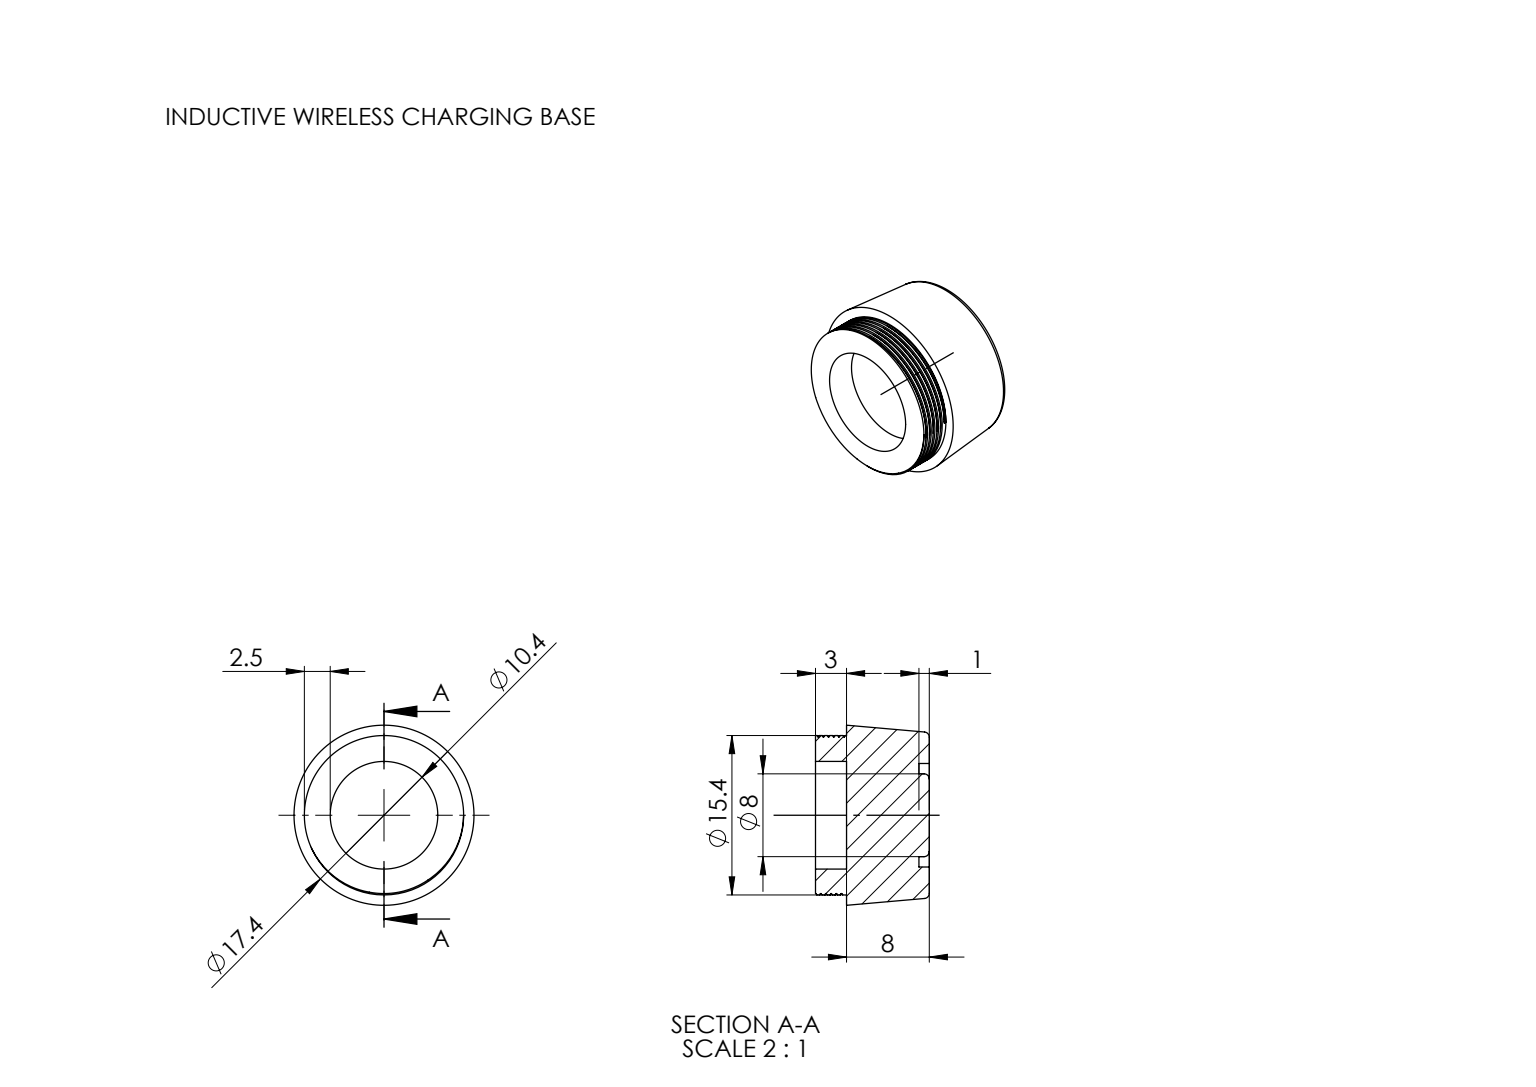
ISO-10303-21;
HEADER;
FILE_DESCRIPTION (('STEP AP214'),
    '1' );
FILE_NAME ('Inductive Wireless Charging Base.step',
    '2026-10-02T09:26:43',
    ( '' ),
    ( '' ),
    'SwSTEP 2.0',
    'SolidWorks 2026',
    '' );
FILE_SCHEMA (( 'AUTOMOTIVE_DESIGN' ));
ENDSEC;

DATA;
#217=EDGE_CURVE ( 'NONE', #101886, #26135, #31742, .T. ) ;
#447=CARTESIAN_POINT ( 'NONE',  ( 186.9479166673494603, -6.668395609140176816, -3.850000000000003642 ) ) ;
#539=ORIENTED_EDGE ( 'NONE', *, *, #28756, .T. ) ;
#549=CARTESIAN_POINT ( 'NONE',  ( 195.0435778713738557, 0.000000000000000000, 0.000000000000000000 ) ) ;
#620=DIRECTION ( 'NONE',  ( 1.000000000000000000, -0.000000000000000000, -0.000000000000000000 ) ) ;
#637=CARTESIAN_POINT ( 'NONE',  ( 184.5000000000000000, 9.429780353434619030E-16, 7.699999999999999289 ) ) ;
#712=CARTESIAN_POINT ( 'NONE',  ( 186.8229166673494603, -4.445597072760107515, 7.700000000000023270 ) ) ;
#800=CARTESIAN_POINT ( 'NONE',  ( 185.5833333333333144, -6.668395609140180369, 3.849999999999994760 ) ) ;
#962=ADVANCED_FACE ( 'NONE', ( #75850 ), #18220, .T. ) ;
#1082=ORIENTED_EDGE ( 'NONE', *, *, #3024, .T. ) ;
#1108=CARTESIAN_POINT ( 'NONE',  ( 185.4062500006828316, -8.891194145520236347, -1.633285867636356693E-15 ) ) ;
#1307=VERTEX_POINT ( 'NONE', #129199 ) ;
#1386=ORIENTED_EDGE ( 'NONE', *, *, #66111, .T. ) ;
#1422=ORIENTED_EDGE ( 'NONE', *, *, #217, .F. ) ;
#1430=FACE_OUTER_BOUND ( 'NONE', #106469, .T. ) ;
#1536=CARTESIAN_POINT ( 'NONE',  ( 184.2552083336747444, 6.551208109652275624, -3.782341765624998686 ) ) ;
#1617=DIRECTION ( 'NONE',  ( -0.9961946980917455452, -1.067350013832299517E-17, 0.08715574274765836016 ) ) ;
#1685=FACE_OUTER_BOUND ( 'NONE', #10697, .T. ) ;
#1745=CARTESIAN_POINT ( 'NONE',  ( 187.1510416670080303, 4.367472073101518859, -7.564683531249999149 ) ) ;
#1928=CARTESIAN_POINT ( 'NONE',  ( 185.4583333333333144, 4.445597072760117285, 7.699999999999999289 ) ) ;
#2069=CARTESIAN_POINT ( 'NONE',  ( 184.5000000000000000, 0.000000000000000000, 0.000000000000000000 ) ) ;
#2080=CARTESIAN_POINT ( 'NONE',  ( 187.3802083336747444, 4.367472073101515306, 7.564683531250000925 ) ) ;
#2130=ORIENTED_EDGE ( 'NONE', *, *, #61987, .T. ) ;
#2172=CARTESIAN_POINT ( 'NONE',  ( 184.3177083336747160, 4.367472073101515306, 7.564683531250000925 ) ) ;
#2331=CIRCLE ( 'NONE', #62997, 4.000000000000000000 ) ;
#2375=CARTESIAN_POINT ( 'NONE',  ( 183.9895833340161175, -4.445597072760115509, -7.700000000000001954 ) ) ;
#2389=CIRCLE ( 'NONE', #63058, 5.200000000000000178 ) ;
#2406=ORIENTED_EDGE ( 'NONE', *, *, #28810, .F. ) ;
#2444=CARTESIAN_POINT ( 'NONE',  ( 184.4999999999999432, -6.631591114337888726, -3.783919631704756092 ) ) ;
#2677=CARTESIAN_POINT ( 'NONE',  ( 184.5000000000000000, -6.267304879582558996, 4.236192450104883100 ) ) ;
#2707=CIRCLE ( 'NONE', #19432, 0.5000000000000000000 ) ;
#2714=ORIENTED_EDGE ( 'NONE', *, *, #127995, .F. ) ;
#2728=CARTESIAN_POINT ( 'NONE',  ( 187.2968750003414300, 8.734944146203032389, 5.348610694689227483E-16 ) ) ;
#2762=EDGE_CURVE ( 'NONE', #109689, #101886, #108407, .T. ) ;
#2828=CARTESIAN_POINT ( 'NONE',  ( 184.4427083336747160, -6.551208109652278289, 3.782341765624995134 ) ) ;
#2996=CARTESIAN_POINT ( 'NONE',  ( 186.0260416670080588, -6.551208109652273848, -3.782341765625003571 ) ) ;
#3024=EDGE_CURVE ( 'NONE', #82135, #52320, #124030, .T. ) ;
#3058=CARTESIAN_POINT ( 'NONE',  ( 185.7395833340161460, 4.445597072760117285, 7.699999999999999289 ) ) ;
#3067=AXIS2_PLACEMENT_3D ( 'NONE', #28494, #69048, #99815 ) ;
#3198=FACE_OUTER_BOUND ( 'NONE', #16127, .T. ) ;
#3309=VERTEX_POINT ( 'NONE', #34058 ) ;
#3320=VECTOR ( 'NONE', #123485, 1000.000000000000000 ) ;
#3378=CARTESIAN_POINT ( 'NONE',  ( 185.1718750003414016, 9.264065473108010111E-16, -7.564683531250000925 ) ) ;
#3380=CARTESIAN_POINT ( 'NONE',  ( 186.4635416670080872, -4.367472073101520635, 7.564683531249999149 ) ) ;
#3429=EDGE_CURVE ( 'NONE', #67593, #79758, #78909, .T. ) ;
#3467=CARTESIAN_POINT ( 'NONE',  ( 184.8333333333333144, 6.668395609140177704, -3.849999999999998312 ) ) ;
#3536=CYLINDRICAL_SURFACE ( 'NONE', #4210, 7.699999999999999289 ) ;
#3631=CARTESIAN_POINT ( 'NONE',  ( 185.2760416670080588, 6.551208109652274736, 3.782341765625001351 ) ) ;
#3634=CARTESIAN_POINT ( 'NONE',  ( 186.1666666666666856, -6.668395609140176816, -3.850000000000003642 ) ) ;
#3688=CARTESIAN_POINT ( 'NONE',  ( 184.4062500006828316, -8.891194145520236347, -1.633285867636356693E-15 ) ) ;
#3819=ORIENTED_EDGE ( 'NONE', *, *, #38635, .F. ) ;
#4014=CARTESIAN_POINT ( 'NONE',  ( 186.4635416670080872, -4.367472073101519747, 7.564683531249999149 ) ) ;
#4049=CARTESIAN_POINT ( 'NONE',  ( 185.9843750003414016, -8.734944146203032389, -1.604583208406767949E-15 ) ) ;
#4097=AXIS2_PLACEMENT_3D ( 'NONE', #10032, #70886, #21131 ) ;
#4210=AXIS2_PLACEMENT_3D ( 'NONE', #73550, #21906, #33647 ) ;
#4252=CARTESIAN_POINT ( 'NONE',  ( 184.5677083336747444, -4.367472073101514418, -7.564683531250002702 ) ) ;
#4305=CARTESIAN_POINT ( 'NONE',  ( 186.3593750003414016, 0.000000000000000000, 7.564683531250000925 ) ) ;
#4364=CARTESIAN_POINT ( 'NONE',  ( 184.5000000000000000, -2.986254062820097310, -7.097343634930640022 ) ) ;
#4463=DIRECTION ( 'NONE',  ( 0.000000000000000000, -1.000000000000000000, 0.000000000000000000 ) ) ;
#4514=APPLICATION_CONTEXT ( 'automotive_design' ) ;
#4558=CIRCLE ( 'NONE', #94463, 3.500000000000000000 ) ;
#4639=CARTESIAN_POINT ( 'NONE',  ( 186.7552083336747444, 6.551208109652275624, -3.782341765624998686 ) ) ;
#4640=CARTESIAN_POINT ( 'NONE',  ( 184.9635416670080588, -4.367472073101520635, 7.564683531249999149 ) ) ;
#4674=CARTESIAN_POINT ( 'NONE',  ( 185.8177083336747160, 4.367472073101515306, 7.564683531250000925 ) ) ;
#4788=CARTESIAN_POINT ( 'NONE',  ( 185.6562500006828031, 8.891194145520236347, 5.444286225454521982E-16 ) ) ;
#4904=CARTESIAN_POINT ( 'NONE',  ( 186.1510416670080588, 4.367472073101518859, -7.564683531249999149 ) ) ;
#4922=CARTESIAN_POINT ( 'NONE',  ( 184.5000000000000000, 9.429780353434619030E-16, 7.699999999999999289 ) ) ;
#4934=ADVANCED_FACE ( 'NONE', ( #116853, #38319 ), #87392, .F. ) ;
#4962=CARTESIAN_POINT ( 'NONE',  ( 185.6093750003413732, 9.264065473108010111E-16, -7.564683531250000925 ) ) ;
#5039=EDGE_LOOP ( 'NONE', ( #7533, #54215, #19907, #25528 ) ) ;
#5109=LINE ( 'NONE', #44402, #37228 ) ;
#5301=CARTESIAN_POINT ( 'NONE',  ( 186.0885416670080872, -6.551208109652273848, -3.782341765625003571 ) ) ;
#5338=CARTESIAN_POINT ( 'NONE',  ( 186.6510416670080872, 4.367472073101518859, -7.564683531249999149 ) ) ;
#5433=AXIS2_PLACEMENT_3D ( 'NONE', #62822, #113189, #13043 ) ;
#5554=CARTESIAN_POINT ( 'NONE',  ( 184.6093750003413732, 9.264065473108010111E-16, -7.564683531250000925 ) ) ;
#5599=CARTESIAN_POINT ( 'NONE',  ( 186.6093750003414016, 9.264065473108010111E-16, -7.564683531250000925 ) ) ;
#5637=ADVANCED_FACE ( 'NONE', ( #22398 ), #110953, .T. ) ;
#5816=( BOUNDED_CURVE ( )  B_SPLINE_CURVE ( 2, ( #29457, #100130, #79209, #128311, #69359, #11079, #128967 ),
 .UNSPECIFIED., .F., .F. ) 
 B_SPLINE_CURVE_WITH_KNOTS ( ( 3, 2, 2, 3 ),
 ( 0.2142857142857144681, 0.2380952380952383041, 0.2619047619047621955, 0.2857142857142859760 ),
 .UNSPECIFIED. ) 
 CURVE ( )  GEOMETRIC_REPRESENTATION_ITEM ( )  RATIONAL_B_SPLINE_CURVE ( ( 0.9999999999999988898, 0.8660254037844397068, 1.000000000000000000, 0.8660254037844387076, 1.000000000000000000, 0.8660254037844371533, 1.000000000000001554 ) ) 
 REPRESENTATION_ITEM ( '' )  );
#5905=CARTESIAN_POINT ( 'NONE',  ( 186.1145833340161175, 6.668395609140177704, -3.849999999999998312 ) ) ;
#5938=CARTESIAN_POINT ( 'NONE',  ( 186.1718750003414016, 9.264065473108010111E-16, -7.564683531250000925 ) ) ;
#5942=CARTESIAN_POINT ( 'NONE',  ( 186.0885416670080872, -6.551208109652273848, -3.782341765625003571 ) ) ;
#5974=CARTESIAN_POINT ( 'NONE',  ( 187.0677083336747160, -4.367472073101514418, -7.564683531250002702 ) ) ;
#6078=EDGE_CURVE ( 'NONE', #70723, #109689, #72930, .T. ) ;
#6192=CARTESIAN_POINT ( 'NONE',  ( 186.7135416670080872, 4.367472073101518859, -7.564683531249999149 ) ) ;
#6220=DIRECTION ( 'NONE',  ( 1.000000000000000000, -0.000000000000000000, -0.000000000000000000 ) ) ;
#6242=CARTESIAN_POINT ( 'NONE',  ( 186.8177083336747160, 4.367472073101515306, 7.564683531250000925 ) ) ;
#6511=DIRECTION ( 'NONE',  ( 1.000000000000000000, -0.000000000000000000, -0.000000000000000000 ) ) ;
#6564=CARTESIAN_POINT ( 'NONE',  ( 186.2916666666666856, 4.445597072760120838, -7.699999999999998401 ) ) ;
#6567=CARTESIAN_POINT ( 'NONE',  ( 185.7552083336747444, 6.551208109652275624, -3.782341765624998686 ) ) ;
#6572=CARTESIAN_POINT ( 'NONE',  ( 185.5312500006828031, 9.429780353434619030E-16, -7.700000000000000178 ) ) ;
#6595=CARTESIAN_POINT ( 'NONE',  ( 186.5260416670080588, -6.551208109652273848, -3.782341765625003571 ) ) ;
#6778=CARTESIAN_POINT ( 'NONE',  ( 187.1562500006828316, 8.891194145520236347, 5.444286225454521982E-16 ) ) ;
#6822=CARTESIAN_POINT ( 'NONE',  ( 185.4635416670080872, -4.367472073101519747, 7.564683531249999149 ) ) ;
#6868=DIRECTION ( 'NONE',  ( 0.4999999999999471534, 0.000000000000000000, -0.8660254037844692387 ) ) ;
#6886=VECTOR ( 'NONE', #112552, 1000.000000000000000 ) ;
#6894=CONICAL_SURFACE ( 'NONE', #50847, 8.699999999999999289, 0.08726646259971666819 ) ;
#6996=ADVANCED_FACE ( 'NONE', ( #25441 ), #102718, .F. ) ;
#7002=ADVANCED_FACE ( 'NONE', ( #53002 ), #28446, .T. ) ;
#7213=DIRECTION ( 'NONE',  ( 1.000000000000000000, -0.000000000000000000, -0.000000000000000000 ) ) ;
#7227=CARTESIAN_POINT ( 'NONE',  ( 186.7500000000000000, 9.429780353434619030E-16, -7.700000000000000178 ) ) ;
#7229=CARTESIAN_POINT ( 'NONE',  ( 185.4218750003414016, 0.000000000000000000, 7.564683531250000925 ) ) ;
#7233=AXIS2_PLACEMENT_3D ( 'NONE', #15454, #95322, #24650 ) ;
#7264=CARTESIAN_POINT ( 'NONE',  ( 185.2343750003414016, 8.734944146203032389, 5.348610694689227483E-16 ) ) ;
#7300=PRODUCT ( 'Inductive Wireless Charging Base', 'Inductive Wireless Charging Base', '', ( #106626 ) ) ;
#7328=ORIENTED_EDGE ( 'NONE', *, *, #95250, .F. ) ;
#7489=CARTESIAN_POINT ( 'NONE',  ( 187.1302083336747444, -4.367472073101514418, -7.564683531250002702 ) ) ;
#7533=ORIENTED_EDGE ( 'NONE', *, *, #8218, .F. ) ;
#7612=CARTESIAN_POINT ( 'NONE',  ( 184.7812500006828031, 0.000000000000000000, 7.700000000000000178 ) ) ;
#7681=CARTESIAN_POINT ( 'NONE',  ( 195.5000000000000000, 0.000000000000000000, 0.000000000000000000 ) ) ;
#7852=CARTESIAN_POINT ( 'NONE',  ( 186.1562500006828031, 8.891194145520236347, 5.444286225454521982E-16 ) ) ;
#7853=DIRECTION ( 'NONE',  ( 1.000000000000000000, -0.000000000000000000, -0.000000000000000000 ) ) ;
#7884=CARTESIAN_POINT ( 'NONE',  ( 184.0468750003414300, -8.734944146203032389, -1.604583208406768146E-15 ) ) ;
#7913=CARTESIAN_POINT ( 'NONE',  ( 184.9427083336747160, -6.551208109652278289, 3.782341765624995134 ) ) ;
#8132=CARTESIAN_POINT ( 'NONE',  ( 186.0885416670080872, -6.551208109652273848, -3.782341765625003571 ) ) ;
#8218=EDGE_CURVE ( 'NONE', #121663, #54095, #122867, .T. ) ;
#8279=VERTEX_POINT ( 'NONE', #111079 ) ;
#8417=SHAPE_DEFINITION_REPRESENTATION ( #77351, #18450 ) ;
#8425=CYLINDRICAL_SURFACE ( 'NONE', #64526, 7.699999999999999289 ) ;
#8518=CARTESIAN_POINT ( 'NONE',  ( 184.1302083336747160, -4.367472073101514418, -7.564683531250002702 ) ) ;
#8530=DIRECTION ( 'NONE',  ( 0.000000000000000000, -1.000000000000000000, 0.000000000000000000 ) ) ;
#8546=CARTESIAN_POINT ( 'NONE',  ( 184.5260416670080588, -6.551208109652273848, -3.782341765625003571 ) ) ;
#8563=( NAMED_UNIT ( * ) SI_UNIT ( $, .STERADIAN. ) SOLID_ANGLE_UNIT ( ) );
#8621=DIRECTION ( 'NONE',  ( 1.000000000000000000, -0.000000000000000000, -0.000000000000000000 ) ) ;
#8765=CARTESIAN_POINT ( 'NONE',  ( 185.7135416670080588, 4.367472073101518859, -7.564683531249999149 ) ) ;
#8828=AXIS2_PLACEMENT_3D ( 'NONE', #66133, #7853, #56309 ) ;
#8935=VECTOR ( 'NONE', #81638, 1000.000000000000114 ) ;
#9183=CARTESIAN_POINT ( 'NONE',  ( 183.9218750003414016, 0.000000000000000000, 7.564683531250000925 ) ) ;
#9449=AXIS2_PLACEMENT_3D ( 'NONE', #93952, #25854, #122764 ) ;
#9462=PRESENTATION_STYLE_ASSIGNMENT (( #69663 ) ) ;
#9826=CARTESIAN_POINT ( 'NONE',  ( 184.6666666666666856, -6.668395609140176816, -3.850000000000003642 ) ) ;
#9879=( NAMED_UNIT ( * ) PLANE_ANGLE_UNIT ( ) SI_UNIT ( $, .RADIAN. ) );
#9972=DIRECTION ( 'NONE',  ( 0.000000000000000000, 0.000000000000000000, 1.000000000000000000 ) ) ;
#10032=CARTESIAN_POINT ( 'NONE',  ( 184.5000000000000000, 0.000000000000000000, 0.000000000000000000 ) ) ;
#10080=CARTESIAN_POINT ( 'NONE',  ( 185.0468750003414016, -8.734944146203032389, -1.604583208406768146E-15 ) ) ;
#10277=CARTESIAN_POINT ( 'NONE',  ( 184.7083333333333428, -4.445597072760175017, -7.699999999999898037 ) ) ;
#10328=CARTESIAN_POINT ( 'NONE',  ( 187.4609375001707008, 0.000000000000000000, 7.632341765625000107 ) ) ;
#10429=CIRCLE ( 'NONE', #77334, 3.500000000000000000 ) ;
#10611=ORIENTED_EDGE ( 'NONE', *, *, #23625, .T. ) ;
#10644=CARTESIAN_POINT ( 'NONE',  ( 0.000000000000000000, 0.000000000000000000, 0.000000000000000000 ) ) ;
#10666=AXIS2_PLACEMENT_3D ( 'NONE', #58179, #68613, #117052 ) ;
#10697=EDGE_LOOP ( 'NONE', ( #109898, #53620, #81214, #33966 ) ) ;
#10776=( BOUNDED_CURVE ( )  B_SPLINE_CURVE ( 2, ( #120233, #10277, #71122, #69842, #60679, #49569, #120867 ),
 .UNSPECIFIED., .F., .F. ) 
 B_SPLINE_CURVE_WITH_KNOTS ( ( 3, 2, 2, 3 ),
 ( 0.7857142857142862535, 0.8095238095238102005, 0.8333333333333340365, 0.8571428571428578724 ),
 .UNSPECIFIED. ) 
 CURVE ( )  GEOMETRIC_REPRESENTATION_ITEM ( )  RATIONAL_B_SPLINE_CURVE ( ( 0.9999999999999968914, 0.8660254037844418162, 1.000000000000000000, 0.8660254037844387076, 1.000000000000000000, 0.8660254037844343777, 1.000000000000004441 ) ) 
 REPRESENTATION_ITEM ( '' )  );
#10901=CARTESIAN_POINT ( 'NONE',  ( 184.7395833340161460, 4.445597072760117285, 7.699999999999999289 ) ) ;
#10977=VECTOR ( 'NONE', #37893, 1000.000000000000000 ) ;
#11079=CARTESIAN_POINT ( 'NONE',  ( 186.3229166673494319, -4.445597072760092416, 7.700000000000049916 ) ) ;
#11120=ORIENTED_EDGE ( 'NONE', *, *, #103788, .F. ) ;
#11135=ORIENTED_EDGE ( 'NONE', *, *, #44217, .T. ) ;
#11175=CARTESIAN_POINT ( 'NONE',  ( 187.2500000000000000, 9.429780353434619030E-16, -7.700000000000000178 ) ) ;
#11573=CARTESIAN_POINT ( 'NONE',  ( 184.0312500006828031, 9.429780353434619030E-16, -7.700000000000000178 ) ) ;
#11909=CARTESIAN_POINT ( 'NONE',  ( 187.1302083336747444, -4.367472073101514418, -7.564683531250002702 ) ) ;
#11938=CARTESIAN_POINT ( 'NONE',  ( 187.5000000000000000, 0.000000000000000000, 0.000000000000000000 ) ) ;
#11956=CIRCLE ( 'NONE', #53720, 5.200000000000000178 ) ;
#11997=ORIENTED_EDGE ( 'NONE', *, *, #52602, .T. ) ;
#12005=ADVANCED_FACE ( 'NONE', ( #70689 ), #110610, .T. ) ;
#12203=ORIENTED_EDGE ( 'NONE', *, *, #28756, .F. ) ;
#12210=CARTESIAN_POINT ( 'NONE',  ( 185.9895833340161460, -4.445597072760115509, -7.700000000000001954 ) ) ;
#12396=CARTESIAN_POINT ( 'NONE',  ( 185.3333333333333144, 6.668395609140177704, -3.849999999999998312 ) ) ;
#12521=EDGE_CURVE ( 'NONE', #85590, #3309, #75602, .T. ) ;
#12635=CARTESIAN_POINT ( 'NONE',  ( 184.1093750003413732, 9.264065473108010111E-16, -7.564683531250000925 ) ) ;
#12681=EDGE_LOOP ( 'NONE', ( #2406, #115928, #39495, #11120 ) ) ;
#12695=MANIFOLD_SOLID_BREP ( 'Cavity1', #56137 ) ;
#12722=CARTESIAN_POINT ( 'NONE',  ( 185.4166666666666856, 6.668395609140176816, 3.850000000000000977 ) ) ;
#12787=CARTESIAN_POINT ( 'NONE',  ( 186.1927083336747160, 6.551208109652275624, -3.782341765624998686 ) ) ;
#12791=DIRECTION ( 'NONE',  ( 0.000000000000000000, 0.000000000000000000, -1.000000000000000000 ) ) ;
#12828=AXIS2_PLACEMENT_3D ( 'NONE', #77197, #105366, #117737 ) ;
#12837=CARTESIAN_POINT ( 'NONE',  ( 184.3645833340161175, -6.668395609140180369, 3.849999999999994760 ) ) ;
#12926=CARTESIAN_POINT ( 'NONE',  ( 186.5000000000000000, 0.000000000000000000, 7.700000000000000178 ) ) ;
#13043=DIRECTION ( 'NONE',  ( 0.000000000000000000, 0.000000000000000000, -1.000000000000000000 ) ) ;
#13048=CARTESIAN_POINT ( 'NONE',  ( 195.5000000000000000, 0.000000000000000000, 0.000000000000000000 ) ) ;
#13128=VECTOR ( 'NONE', #84395, 1000.000000000000000 ) ;
#13181=CARTESIAN_POINT ( 'NONE',  ( 185.4635416670080872, -4.367472073101519747, 7.564683531249999149 ) ) ;
#13235=CARTESIAN_POINT ( 'NONE',  ( 185.4895833340161175, -4.445597072760163471, -7.699999999999919353 ) ) ;
#13270=CARTESIAN_POINT ( 'NONE',  ( 184.9166666666666856, 6.668395609140176816, 3.850000000000000977 ) ) ;
#13276=CARTESIAN_POINT ( 'NONE',  ( 184.4010416670080872, -4.367472073101519747, 7.564683531249999149 ) ) ;
#13365=ORIENTED_EDGE ( 'NONE', *, *, #41805, .F. ) ;
#13440=CARTESIAN_POINT ( 'NONE',  ( 186.6093750003414016, 9.264065473108010111E-16, -7.564683531250000925 ) ) ;
#13496=CARTESIAN_POINT ( 'NONE',  ( 184.8229166673494603, -4.445597072760122614, 7.699999999999998401 ) ) ;
#13742=PLANE ( 'NONE',  #84182 ) ;
#13832=CARTESIAN_POINT ( 'NONE',  ( 185.7552083336747444, 6.551208109652275624, -3.782341765624998686 ) ) ;
#13836=CARTESIAN_POINT ( 'NONE',  ( 186.2552083336747444, 6.551208109652275624, -3.782341765624998686 ) ) ;
#13869=CARTESIAN_POINT ( 'NONE',  ( 186.0677083336747444, -4.367472073101514418, -7.564683531250002702 ) ) ;
#13916=CARTESIAN_POINT ( 'NONE',  ( 185.8229166673494319, -4.445597072760079982, 7.700000000000070344 ) ) ;
#13972=EDGE_LOOP ( 'NONE', ( #84717, #41693, #92938, #7328 ) ) ;
#14015=CARTESIAN_POINT ( 'NONE',  ( 184.5000000000000000, 0.000000000000000000, -7.699999999999999289 ) ) ;
#14025=ORIENTED_EDGE ( 'NONE', *, *, #34914, .T. ) ;
#14076=CARTESIAN_POINT ( 'NONE',  ( 184.6927083336747160, 6.551208109652275624, -3.782341765624998686 ) ) ;
#14113=AXIS2_PLACEMENT_3D ( 'NONE', #19161, #70228, #72168 ) ;
#14141=CARTESIAN_POINT ( 'NONE',  ( 186.4427083336747160, -6.551208109652278289, 3.782341765624995134 ) ) ;
#14229=( BOUNDED_CURVE ( )  B_SPLINE_CURVE ( 2, ( #60447, #108228, #100354, #68948, #28392, #108860, #18560 ),
 .UNSPECIFIED., .F., .F. ) 
 B_SPLINE_CURVE_WITH_KNOTS ( ( 3, 2, 2, 3 ),
 ( 0.4285714285714289362, 0.4523809523809527722, 0.4761904761904766081, 0.5000000000000004441 ),
 .UNSPECIFIED. ) 
 CURVE ( )  GEOMETRIC_REPRESENTATION_ITEM ( )  RATIONAL_B_SPLINE_CURVE ( ( 0.9999999999999977796, 0.8660254037844409281, 1.000000000000000000, 0.8660254037844387076, 1.000000000000000000, 0.8660254037844361541, 1.000000000000002442 ) ) 
 REPRESENTATION_ITEM ( '' )  );
#14263=CARTESIAN_POINT ( 'NONE',  ( 184.5000000000000000, -2.986254062820097310, -7.097343634930640022 ) ) ;
#14466=CARTESIAN_POINT ( 'NONE',  ( 185.5052083336747444, -6.551208109652278289, 3.782341765624995134 ) ) ;
#14469=CARTESIAN_POINT ( 'NONE',  ( 185.3385416670080872, 6.551208109652274736, 3.782341765625001351 ) ) ;
#14505=CARTESIAN_POINT ( 'NONE',  ( 185.9427083336747160, -6.551208109652278289, 3.782341765624995134 ) ) ;
#14524=CARTESIAN_POINT ( 'NONE',  ( 185.3645833340161175, -6.668395609140180369, 3.849999999999994760 ) ) ;
#14556=CARTESIAN_POINT ( 'NONE',  ( 185.7812500006828031, 0.000000000000000000, 7.700000000000000178 ) ) ;
#14718=CARTESIAN_POINT ( 'NONE',  ( 184.4843750003414016, -8.734944146203032389, -1.604583208406768146E-15 ) ) ;
#14765=CARTESIAN_POINT ( 'NONE',  ( 185.4427083336747160, -6.551208109652278289, 3.782341765624995134 ) ) ;
#14851=ORIENTED_EDGE ( 'NONE', *, *, #51179, .F. ) ;
#15054=CARTESIAN_POINT ( 'NONE',  ( 184.5000000000000000, -7.430520870378829024, -1.418378131116527108 ) ) ;
#15099=CARTESIAN_POINT ( 'NONE',  ( 186.2968750003414584, 8.734944146203032389, 5.348610694689227483E-16 ) ) ;
#15125=AXIS2_PLACEMENT_3D ( 'NONE', #39212, #79121, #69267 ) ;
#15347=DIRECTION ( 'NONE',  ( 1.000000000000000000, -0.000000000000000000, -0.000000000000000000 ) ) ;
#15362=CARTESIAN_POINT ( 'NONE',  ( 185.4010416670080588, -4.367472073101519747, 7.564683531249999149 ) ) ;
#15423=CARTESIAN_POINT ( 'NONE',  ( 185.3177083336747160, 4.367472073101515306, 7.564683531250000925 ) ) ;
#15454=CARTESIAN_POINT ( 'NONE',  ( 187.5000000000000000, 0.000000000000000000, 0.000000000000000000 ) ) ;
#15764=( BOUNDED_CURVE ( )  B_SPLINE_CURVE ( 2, ( #114067, #45339, #24397, #104244, #125176, #13916, #14556 ),
 .UNSPECIFIED., .F., .F. ) 
 B_SPLINE_CURVE_WITH_KNOTS ( ( 3, 2, 2, 3 ),
 ( 0.3571428571428574283, 0.3809523809523812643, 0.4047619047619051003, 0.4285714285714289362 ),
 .UNSPECIFIED. ) 
 CURVE ( )  GEOMETRIC_REPRESENTATION_ITEM ( )  RATIONAL_B_SPLINE_CURVE ( ( 0.9999999999999984457, 0.8660254037844402619, 1.000000000000000000, 0.8660254037844387076, 1.000000000000000000, 0.8660254037844364872, 1.000000000000002220 ) ) 
 REPRESENTATION_ITEM ( '' )  );
#15766=CARTESIAN_POINT ( 'NONE',  ( 185.0468750003414016, -8.734944146203032389, -1.604583208406768146E-15 ) ) ;
#15768=CARTESIAN_POINT ( 'NONE',  ( 184.7552083336747444, 6.551208109652275624, -3.782341765624998686 ) ) ;
#15856=CYLINDRICAL_SURFACE ( 'NONE', #119801, 7.699999999999999289 ) ;
#16013=CARTESIAN_POINT ( 'NONE',  ( 187.0468750003414300, -8.734944146203032389, -1.604583208406768146E-15 ) ) ;
#16053=CARTESIAN_POINT ( 'NONE',  ( 187.3203125005121024, 0.000000000000000000, 7.632341765625000107 ) ) ;
#16063=CARTESIAN_POINT ( 'NONE',  ( 184.8177083336747160, 4.367472073101515306, 7.564683531250000925 ) ) ;
#16127=EDGE_LOOP ( 'NONE', ( #72186, #18546, #55572, #73590 ) ) ;
#16235=EDGE_CURVE ( 'NONE', #82540, #27061, #113643, .T. ) ;
#16266=VERTEX_POINT ( 'NONE', #71255 ) ;
#16302=VECTOR ( 'NONE', #22749, 1000.000000000000000 ) ;
#16352=AXIS2_PLACEMENT_3D ( 'NONE', #121542, #92084, #111063 ) ;
#16377=LINE ( 'NONE', #49760, #90784 ) ;
#16393=CARTESIAN_POINT ( 'NONE',  ( 184.2968750003414300, 8.734944146203032389, 5.348610694689227483E-16 ) ) ;
#16396=CARTESIAN_POINT ( 'NONE',  ( 184.7968750003414584, 8.734944146203032389, 5.348610694689227483E-16 ) ) ;
#16439=ORIENTED_EDGE ( 'NONE', *, *, #59537, .T. ) ;
#16493=CARTESIAN_POINT ( 'NONE',  ( 186.0416666666666572, -4.445597072760079982, 7.700000000000070344 ) ) ;
#16544=EDGE_CURVE ( 'NONE', #82135, #97220, #55161, .T. ) ;
#16564=CARTESIAN_POINT ( 'NONE',  ( 185.1562500006828031, 8.891194145520236347, 5.444286225454521982E-16 ) ) ;
#16597=ORIENTED_EDGE ( 'NONE', *, *, #127995, .T. ) ;
#16634=AXIS2_PLACEMENT_3D ( 'NONE', #98456, #29736, #89298 ) ;
#16653=CARTESIAN_POINT ( 'NONE',  ( 185.8802083336747444, 4.367472073101515306, 7.564683531250000925 ) ) ;
#16681=ORIENTED_EDGE ( 'NONE', *, *, #19986, .T. ) ;
#16705=CARTESIAN_POINT ( 'NONE',  ( 185.2760416670080588, 6.551208109652274736, 3.782341765625001351 ) ) ;
#16770=CARTESIAN_POINT ( 'NONE',  ( 184.8645833340161175, -6.668395609140180369, 3.849999999999994760 ) ) ;
#16906=LINE ( 'NONE', #56213, #13128 ) ;
#16967=ORIENTED_EDGE ( 'NONE', *, *, #44217, .F. ) ;
#17023=CARTESIAN_POINT ( 'NONE',  ( 187.3333333333333144, 6.668395609140177704, -3.849999999999998312 ) ) ;
#17060=CARTESIAN_POINT ( 'NONE',  ( 184.6927083336747160, 6.551208109652275624, -3.782341765624998686 ) ) ;
#17088=AXIS2_PLACEMENT_3D ( 'NONE', #35751, #56016, #84842 ) ;
#17116=CARTESIAN_POINT ( 'NONE',  ( 186.2083333333333428, -4.445597072760145707, -7.699999999999951328 ) ) ;
#17152=PLANE ( 'NONE',  #67341 ) ;
#17161=EDGE_LOOP ( 'NONE', ( #107186, #36476, #78326, #49216 ) ) ;
#17287=CARTESIAN_POINT ( 'NONE',  ( 187.0052083336747444, -6.551208109652278289, 3.782341765624995134 ) ) ;
#17311=( NAMED_UNIT ( * ) SI_UNIT ( $, .STERADIAN. ) SOLID_ANGLE_UNIT ( ) );
#17430=VERTEX_POINT ( 'NONE', #63251 ) ;
#17526=CARTESIAN_POINT ( 'NONE',  ( 184.5000000000000000, 0.000000000000000000, -7.699999999999999289 ) ) ;
#17533=VERTEX_POINT ( 'NONE', #113644 ) ;
#17699=CARTESIAN_POINT ( 'NONE',  ( 187.0000000000000000, 0.000000000000000000, 7.700000000000000178 ) ) ;
#17958=CARTESIAN_POINT ( 'NONE',  ( 186.6302083336747160, -4.367472073101514418, -7.564683531250002702 ) ) ;
#17985=EDGE_CURVE ( 'NONE', #16266, #22601, #54816, .T. ) ;
#18154=CYLINDRICAL_SURFACE ( 'NONE', #58923, 7.699999999999999289 ) ;
#18157=AXIS2_PLACEMENT_3D ( 'NONE', #2069, #99647, #9972 ) ;
#18170=CARTESIAN_POINT ( 'NONE',  ( 187.0312500006828031, 9.429780353434619030E-16, -7.700000000000000178 ) ) ;
#18183=ADVANCED_FACE ( 'NONE', ( #90960 ), #73600, .T. ) ;
#18220=CYLINDRICAL_SURFACE ( 'NONE', #10666, 4.000000000000000000 ) ;
#18355=CARTESIAN_POINT ( 'NONE',  ( 186.4583333333333144, 4.445597072760117285, 7.699999999999999289 ) ) ;
#18360=DIRECTION ( 'NONE',  ( 0.000000000000000000, 0.000000000000000000, -1.000000000000000000 ) ) ;
#18383=CARTESIAN_POINT ( 'NONE',  ( 185.6510416670080303, 4.367472073101518859, -7.564683531249999149 ) ) ;
#18450=SHAPE_REPRESENTATION ( 'Inductive Wireless Charging Base', ( #108296 ), #37304 ) ;
#18546=ORIENTED_EDGE ( 'NONE', *, *, #92244, .T. ) ;
#18556=CYLINDRICAL_SURFACE ( 'NONE', #4097, 7.699999999999999289 ) ;
#18560=CARTESIAN_POINT ( 'NONE',  ( 185.7500000000000000, 9.429780353434619030E-16, -7.700000000000000178 ) ) ;
#18606=CARTESIAN_POINT ( 'NONE',  ( 186.1718750003414016, 9.264065473108010111E-16, -7.564683531250000925 ) ) ;
#18625=ORIENTED_EDGE ( 'NONE', *, *, #3429, .T. ) ;
#18668=CYLINDRICAL_SURFACE ( 'NONE', #29927, 7.699999999999999289 ) ;
#18741=CARTESIAN_POINT ( 'NONE',  ( 184.5000000000000000, 0.000000000000000000, -5.200000000000000178 ) ) ;
#18816=FACE_OUTER_BOUND ( 'NONE', #18940, .T. ) ;
#18885=DIRECTION ( 'NONE',  ( -1.000000000000000000, -0.000000000000000000, -0.000000000000000000 ) ) ;
#18940=EDGE_LOOP ( 'NONE', ( #91829, #58214, #34205, #82778, #48164, #34402, #69224, #118172, #104712, #13365, #90243, #89668, #112364, #60147, #77509 ) ) ;
#18987=CARTESIAN_POINT ( 'NONE',  ( 185.5000000000000000, 0.000000000000000000, 7.700000000000000178 ) ) ;
#19017=CARTESIAN_POINT ( 'NONE',  ( 185.5677083336747160, -4.367472073101514418, -7.564683531250002702 ) ) ;
#19026=ORIENTED_EDGE ( 'NONE', *, *, #16544, .F. ) ;
#19126=ORIENTED_EDGE ( 'NONE', *, *, #38452, .T. ) ;
#19131=CARTESIAN_POINT ( 'NONE',  ( 185.6249999999999716, -8.891194145520236347, -1.633285867636356299E-15 ) ) ;
#19161=CARTESIAN_POINT ( 'NONE',  ( 184.5000000000000000, 0.000000000000000000, 0.000000000000000000 ) ) ;
#19258=FILL_AREA_STYLE ('',( #127308 ) ) ;
#19263=ORIENTED_EDGE ( 'NONE', *, *, #217, .T. ) ;
#19371=CARTESIAN_POINT ( 'NONE',  ( 186.5000000000000000, 0.000000000000000000, 7.700000000000000178 ) ) ;
#19390=CARTESIAN_POINT ( 'NONE',  ( 186.9427083336747160, -6.551208109652278289, 3.782341765624995134 ) ) ;
#19432=AXIS2_PLACEMENT_3D ( 'NONE', #110698, #41346, #43278 ) ;
#19522=ORIENTED_EDGE ( 'NONE', *, *, #23625, .F. ) ;
#19629=AXIS2_PLACEMENT_3D ( 'NONE', #101705, #80784, #90578 ) ;
#19654=CARTESIAN_POINT ( 'NONE',  ( 184.6250000000000000, -8.891194145520236347, -1.633285867636356693E-15 ) ) ;
#19783=CIRCLE ( 'NONE', #7233, 7.699999999999999289 ) ;
#19907=ORIENTED_EDGE ( 'NONE', *, *, #42280, .T. ) ;
#19973=CARTESIAN_POINT ( 'NONE',  ( 187.5000000000000000, 0.000000000000000000, 0.000000000000000000 ) ) ;
#19986=EDGE_CURVE ( 'NONE', #67674, #17430, #103413, .T. ) ;
#20101=CARTESIAN_POINT ( 'NONE',  ( 184.5000000000000000, 6.368163355566236381E-16, 5.200000000000000178 ) ) ;
#20115=CARTESIAN_POINT ( 'NONE',  ( 186.5312500006828031, 9.429780353434619030E-16, -7.700000000000000178 ) ) ;
#20195=CARTESIAN_POINT ( 'NONE',  ( 195.5000000000000000, 4.592425496802573972E-16, 3.500000000000000000 ) ) ;
#20294=CARTESIAN_POINT ( 'NONE',  ( 184.7500000000000000, 9.429780353434619030E-16, -7.700000000000000178 ) ) ;
#20525=ADVANCED_FACE ( 'NONE', ( #36846, #87211 ), #17152, .T. ) ;
#20580=ORIENTED_EDGE ( 'NONE', *, *, #103912, .T. ) ;
#20939=CARTESIAN_POINT ( 'NONE',  ( 185.4166666666666856, 6.668395609140176816, 3.850000000000000977 ) ) ;
#20986=CARTESIAN_POINT ( 'NONE',  ( 195.5000000000000000, 0.000000000000000000, 0.000000000000000000 ) ) ;
#21121=ORIENTED_EDGE ( 'NONE', *, *, #99642, .T. ) ;
#21131=DIRECTION ( 'NONE',  ( 0.000000000000000000, 0.000000000000000000, -1.000000000000000000 ) ) ;
#21334=ADVANCED_FACE ( 'NONE', ( #63311 ), #67536, .T. ) ;
#21386=EDGE_LOOP ( 'NONE', ( #52495, #36854 ) ) ;
#21392=CARTESIAN_POINT ( 'NONE',  ( 184.8645833340161175, -6.668395609140180369, 3.849999999999994760 ) ) ;
#21492=DIRECTION ( 'NONE',  ( -1.000000000000000000, -0.000000000000000000, -0.000000000000000000 ) ) ;
#21524=ORIENTED_EDGE ( 'NONE', *, *, #41000, .T. ) ;
#21772=CARTESIAN_POINT ( 'NONE',  ( 195.5000000000000000, 0.000000000000000000, -3.500000000000000000 ) ) ;
#21850=CARTESIAN_POINT ( 'NONE',  ( 184.3385416670080872, 6.551208109652274736, 3.782341765625001351 ) ) ;
#21906=DIRECTION ( 'NONE',  ( 1.000000000000000000, -0.000000000000000000, -0.000000000000000000 ) ) ;
#22062=CARTESIAN_POINT ( 'NONE',  ( 183.9479166673494603, -6.668395609140176816, -3.850000000000003642 ) ) ;
#22366=CARTESIAN_POINT ( 'NONE',  ( 187.1666666666666856, -6.668395609140176816, -3.850000000000003642 ) ) ;
#22398=FACE_OUTER_BOUND ( 'NONE', #35561, .T. ) ;
#22442=ORIENTED_EDGE ( 'NONE', *, *, #92244, .F. ) ;
#22459=ORIENTED_EDGE ( 'NONE', *, *, #67561, .T. ) ;
#22519=DIRECTION ( 'NONE',  ( 1.000000000000000000, 0.000000000000000000, 0.000000000000000000 ) ) ;
#22582=DIRECTION ( 'NONE',  ( 0.000000000000000000, 0.000000000000000000, 1.000000000000000000 ) ) ;
#22601=VERTEX_POINT ( 'NONE', #20195 ) ;
#22646=CARTESIAN_POINT ( 'NONE',  ( 186.2343750003414016, 8.734944146203032389, 5.348610694689227483E-16 ) ) ;
#22652=CARTESIAN_POINT ( 'NONE',  ( 184.5000000000000000, 0.000000000000000000, 0.000000000000000000 ) ) ;
#22670=ORIENTED_EDGE ( 'NONE', *, *, #6078, .F. ) ;
#22707=CARTESIAN_POINT ( 'NONE',  ( 185.7812500006828031, 0.000000000000000000, 7.700000000000000178 ) ) ;
#22749=DIRECTION ( 'NONE',  ( 1.000000000000000000, -0.000000000000000000, -0.000000000000000000 ) ) ;
#22767=ORIENTED_EDGE ( 'NONE', *, *, #47594, .T. ) ;
#22943=ORIENTED_EDGE ( 'NONE', *, *, #125058, .T. ) ;
#23028=CARTESIAN_POINT ( 'NONE',  ( 186.7968750003414300, 8.734944146203032389, 5.348610694689227483E-16 ) ) ;
#23030=CARTESIAN_POINT ( 'NONE',  ( 186.7135416670080872, 4.367472073101518859, -7.564683531249999149 ) ) ;
#23080=CARTESIAN_POINT ( 'NONE',  ( 185.4062500006828031, -8.891194145520236347, -1.633285867636356299E-15 ) ) ;
#23115=CARTESIAN_POINT ( 'NONE',  ( 195.0435778713738557, 0.000000000000000000, 0.000000000000000000 ) ) ;
#23257=CARTESIAN_POINT ( 'NONE',  ( 185.9843750003414016, -8.734944146203032389, -1.604583208406768146E-15 ) ) ;
#23316=CARTESIAN_POINT ( 'NONE',  ( 185.6145833340161175, 6.668395609140177704, -3.849999999999998312 ) ) ;
#23428=AXIS2_PLACEMENT_3D ( 'NONE', #100141, #39937, #120421 ) ;
#23577=CARTESIAN_POINT ( 'NONE',  ( 186.5833333333333144, -6.668395609140180369, 3.849999999999994760 ) ) ;
#23625=EDGE_CURVE ( 'NONE', #121663, #50143, #96054, .T. ) ;
#23667=CARTESIAN_POINT ( 'NONE',  ( 186.0468750003414300, -8.734944146203032389, -1.604583208406768146E-15 ) ) ;
#23670=CARTESIAN_POINT ( 'NONE',  ( 186.4218750003414016, 0.000000000000000000, 7.564683531250000925 ) ) ;
#23693=CARTESIAN_POINT ( 'NONE',  ( 184.7500000000000000, 9.429780353434619030E-16, -7.700000000000000178 ) ) ;
#23726=EDGE_CURVE ( 'NONE', #70184, #91613, #15764, .T. ) ;
#23906=LINE ( 'NONE', #116131, #94190 ) ;
#23930=CARTESIAN_POINT ( 'NONE',  ( 184.8177083336747160, 4.367472073101515306, 7.564683531250000925 ) ) ;
#23985=CARTESIAN_POINT ( 'NONE',  ( 185.8229166673494319, -4.445597072760122614, 7.699999999999998401 ) ) ;
#24048=CARTESIAN_POINT ( 'NONE',  ( 184.5000000000000000, -7.430520870378829024, -1.418378131116527108 ) ) ;
#24195=( BOUNDED_CURVE ( )  B_SPLINE_CURVE ( 2, ( #69447, #104079, #92314, #61593, #23577, #113907, #43886 ),
 .UNSPECIFIED., .F., .F. ) 
 B_SPLINE_CURVE_WITH_KNOTS ( ( 3, 2, 2, 3 ),
 ( 0.2142857142857144681, 0.2380952380952383041, 0.2619047619047621955, 0.2857142857142859760 ),
 .UNSPECIFIED. ) 
 CURVE ( )  GEOMETRIC_REPRESENTATION_ITEM ( )  RATIONAL_B_SPLINE_CURVE ( ( 0.9999999999999988898, 0.8660254037844397068, 1.000000000000000000, 0.8660254037844387076, 1.000000000000000000, 0.8660254037844371533, 1.000000000000001554 ) ) 
 REPRESENTATION_ITEM ( '' )  );
#24311=CARTESIAN_POINT ( 'NONE',  ( 185.7135416670080588, 4.367472073101518859, -7.564683531249999149 ) ) ;
#24314=CARTESIAN_POINT ( 'NONE',  ( 184.5052083336747444, -6.551208109652278289, 3.782341765624995134 ) ) ;
#24367=CARTESIAN_POINT ( 'NONE',  ( 186.9583333333332860, 4.445597072760133273, 7.699999999999975309 ) ) ;
#24387=ADVANCED_FACE ( 'NONE', ( #71742 ), #111669, .T. ) ;
#24397=CARTESIAN_POINT ( 'NONE',  ( 185.9479166673494603, -6.668395609140176816, -3.850000000000003642 ) ) ;
#24402=CARTESIAN_POINT ( 'NONE',  ( 184.0260416670080588, -6.551208109652273848, -3.782341765625003571 ) ) ;
#24494=CARTESIAN_POINT ( 'NONE',  ( 187.5000000000000000, 6.368163355566236381E-16, 5.200000000000000178 ) ) ;
#24562=CARTESIAN_POINT ( 'NONE',  ( 185.2343750003414016, 8.734944146203032389, 5.348610694689227483E-16 ) ) ;
#24628=CARTESIAN_POINT ( 'NONE',  ( 185.5260416670080588, -6.551208109652273848, -3.782341765625003571 ) ) ;
#24650=DIRECTION ( 'NONE',  ( 0.000000000000000000, 0.000000000000000000, 1.000000000000000000 ) ) ;
#24746=ADVANCED_FACE ( 'NONE', ( #28445 ), #6894, .T. ) ;
#24847=EDGE_LOOP ( 'NONE', ( #26293, #12203, #62356, #41695 ) ) ;
#24888=DIRECTION ( 'NONE',  ( 0.000000000000000000, 0.000000000000000000, -1.000000000000000000 ) ) ;
#24954=CARTESIAN_POINT ( 'NONE',  ( 185.3385416670080872, 6.551208109652274736, 3.782341765625001351 ) ) ;
#25194=CARTESIAN_POINT ( 'NONE',  ( 186.7343750003414300, 8.734944146203032389, 5.348610694689227483E-16 ) ) ;
#25243=CARTESIAN_POINT ( 'NONE',  ( 186.9010416670080303, -4.367472073101519747, 7.564683531249999149 ) ) ;
#25303=EDGE_CURVE ( 'NONE', #97440, #36662, #29179, .T. ) ;
#25353=EDGE_LOOP ( 'NONE', ( #60289, #68706, #43931, #107555 ) ) ;
#25441=FACE_OUTER_BOUND ( 'NONE', #46842, .T. ) ;
#25458=EDGE_CURVE ( 'NONE', #52063, #55284, #69281, .T. ) ;
#25494=DIRECTION ( 'NONE',  ( 0.000000000000000000, 0.000000000000000000, -1.000000000000000000 ) ) ;
#25528=ORIENTED_EDGE ( 'NONE', *, *, #40311, .T. ) ;
#25562=AXIS2_PLACEMENT_3D ( 'NONE', #26880, #43474, #53925 ) ;
#25582=CARTESIAN_POINT ( 'NONE',  ( 185.2552083336747444, 6.551208109652275624, -3.782341765624998686 ) ) ;
#25584=CARTESIAN_POINT ( 'NONE',  ( 185.6718750003414016, 9.264065473108010111E-16, -7.564683531250000925 ) ) ;
#25617=CARTESIAN_POINT ( 'NONE',  ( 186.4010416670080588, -4.367472073101520635, 7.564683531249999149 ) ) ;
#25717=DIRECTION ( 'NONE',  ( 1.000000000000000000, 0.000000000000000000, 0.000000000000000000 ) ) ;
#25840=ADVANCED_BREP_SHAPE_REPRESENTATION ( '', ( #12695, #108296 ), #37304 ) ;
#25854=DIRECTION ( 'NONE',  ( 1.000000000000000000, 0.000000000000000000, 0.000000000000000000 ) ) ;
#25855=CARTESIAN_POINT ( 'NONE',  ( 187.4218750003414016, 0.000000000000000000, 7.564683531250000925 ) ) ;
#25915=CARTESIAN_POINT ( 'NONE',  ( 185.1927083336747160, 6.551208109652275624, -3.782341765624998686 ) ) ;
#25927=ADVANCED_FACE ( 'NONE', ( #55560 ), #105942, .T. ) ;
#25985=CIRCLE ( 'NONE', #120067, 0.4999999999999995559 ) ;
#26068=EDGE_CURVE ( 'NONE', #87604, #65296, #107227, .T. ) ;
#26076=DIRECTION ( 'NONE',  ( -1.000000000000000000, 0.000000000000000000, 0.000000000000000000 ) ) ;
#26135=VERTEX_POINT ( 'NONE', #24494 ) ;
#26254=CARTESIAN_POINT ( 'NONE',  ( 186.5416666666666856, -4.445597072760122614, 7.699999999999998401 ) ) ;
#26256=CARTESIAN_POINT ( 'NONE',  ( 186.0052083336747444, -6.551208109652278289, 3.782341765624995134 ) ) ;
#26293=ORIENTED_EDGE ( 'NONE', *, *, #17985, .F. ) ;
#26507=CARTESIAN_POINT ( 'NONE',  ( 186.1302083336747444, -4.367472073101514418, -7.564683531250002702 ) ) ;
#26558=CARTESIAN_POINT ( 'NONE',  ( 185.6927083336747160, 6.551208109652275624, -3.782341765624998686 ) ) ;
#26753=ORIENTED_EDGE ( 'NONE', *, *, #42280, .F. ) ;
#26880=CARTESIAN_POINT ( 'NONE',  ( 195.0000000000000000, 4.286263797015736595E-16, 3.500000000000000000 ) ) ;
#26893=CARTESIAN_POINT ( 'NONE',  ( 187.0833333333333144, -6.668395609140180369, 3.849999999999994760 ) ) ;
#26924=CARTESIAN_POINT ( 'NONE',  ( 185.3593750003413732, 0.000000000000000000, 7.564683531250000925 ) ) ;
#27061=VERTEX_POINT ( 'NONE', #58957 ) ;
#27102=CARTESIAN_POINT ( 'NONE',  ( 187.0729166673494603, 4.445597072760113733, -7.700000000000009948 ) ) ;
#27144=CARTESIAN_POINT ( 'NONE',  ( 183.9427083336747160, -6.551208109652278289, 3.782341765624995134 ) ) ;
#27415=EDGE_CURVE ( 'NONE', #3309, #35519, #100267, .T. ) ;
#27417=CARTESIAN_POINT ( 'NONE',  ( 184.5000000000000000, 0.000000000000000000, 0.000000000000000000 ) ) ;
#27433=CARTESIAN_POINT ( 'NONE',  ( 185.0833333333333144, -6.668395609140180369, 3.849999999999994760 ) ) ;
#27481=FACE_OUTER_BOUND ( 'NONE', #121551, .T. ) ;
#27511=CARTESIAN_POINT ( 'NONE',  ( 186.0833333333333144, -6.668395609140180369, 3.849999999999994760 ) ) ;
#27677=EDGE_CURVE ( 'NONE', #99122, #99741, #2331, .T. ) ;
#27772=CARTESIAN_POINT ( 'NONE',  ( 185.8385416670080872, 6.551208109652274736, 3.782341765625001351 ) ) ;
#28096=CARTESIAN_POINT ( 'NONE',  ( 185.1250000000000000, -8.891194145520236347, -1.633285867636356299E-15 ) ) ;
#28103=AXIS2_PLACEMENT_3D ( 'NONE', #128353, #8530, #48480 ) ;
#28185=CARTESIAN_POINT ( 'NONE',  ( 186.5833333333333144, -6.668395609140180369, 3.849999999999994760 ) ) ;
#28293=CARTESIAN_POINT ( 'NONE',  ( 184.5000000000000000, 0.000000000000000000, 0.000000000000000000 ) ) ;
#28346=CARTESIAN_POINT ( 'NONE',  ( 185.7500000000000000, 9.429780353434619030E-16, -7.700000000000000178 ) ) ;
#28392=CARTESIAN_POINT ( 'NONE',  ( 185.8333333333333144, 6.668395609140177704, -3.849999999999998312 ) ) ;
#28439=CARTESIAN_POINT ( 'NONE',  ( 186.7968750003414300, 8.734944146203032389, 5.348610694689227483E-16 ) ) ;
#28445=FACE_OUTER_BOUND ( 'NONE', #61866, .T. ) ;
#28446=TOROIDAL_SURFACE ( 'NONE', #101599, 3.500000000000000000, 0.5000000000000000000 ) ;
#28460=FACE_BOUND ( 'NONE', #63190, .T. ) ;
#28494=CARTESIAN_POINT ( 'NONE',  ( 187.5000000000000000, 0.000000000000000000, 0.000000000000000000 ) ) ;
#28703=CARTESIAN_POINT ( 'NONE',  ( 186.6145833340161175, 6.668395609140177704, -3.849999999999998312 ) ) ;
#28707=VERTEX_POINT ( 'NONE', #117714 ) ;
#28756=EDGE_CURVE ( 'NONE', #34917, #16266, #29731, .T. ) ;
#28772=CARTESIAN_POINT ( 'NONE',  ( 184.5000000000000000, 0.000000000000000000, 0.000000000000000000 ) ) ;
#28810=EDGE_CURVE ( 'NONE', #16266, #34917, #90360, .T. ) ;
#28837=CARTESIAN_POINT ( 'NONE',  ( 185.5833333333333144, -6.668395609140180369, 3.849999999999994760 ) ) ;
#28843=CARTESIAN_POINT ( 'NONE',  ( 194.5000000000000000, 0.000000000000000000, 0.000000000000000000 ) ) ;
#28868=CARTESIAN_POINT ( 'NONE',  ( 185.5260416670080588, -6.551208109652273848, -3.782341765625003571 ) ) ;
#28970=DIRECTION ( 'NONE',  ( 1.000000000000000000, -0.000000000000000000, -0.000000000000000000 ) ) ;
#29023=CYLINDRICAL_SURFACE ( 'NONE', #14113, 7.699999999999999289 ) ;
#29069=ADVANCED_FACE ( 'NONE', ( #89975 ), #18668, .T. ) ;
#29179=( BOUNDED_CURVE ( )  B_SPLINE_CURVE ( 2, ( #28346, #129144, #39473, #19131, #800, #98348, #59093 ),
 .UNSPECIFIED., .F., .F. ) 
 B_SPLINE_CURVE_WITH_KNOTS ( ( 3, 2, 2, 3 ),
 ( 0.5000000000000004441, 0.5238095238095242800, 0.5476190476190482270, 0.5714285714285719520 ),
 .UNSPECIFIED. ) 
 CURVE ( )  GEOMETRIC_REPRESENTATION_ITEM ( )  RATIONAL_B_SPLINE_CURVE ( ( 0.9999999999999974465, 0.8660254037844412611, 1.000000000000000000, 0.8660254037844387076, 1.000000000000000000, 0.8660254037844355990, 1.000000000000003109 ) ) 
 REPRESENTATION_ITEM ( '' )  );
#29244=CARTESIAN_POINT ( 'NONE',  ( 187.1093750003414016, 9.264065473108010111E-16, -7.564683531250000925 ) ) ;
#29300=CARTESIAN_POINT ( 'NONE',  ( 186.0729166673494319, 4.445597072760120838, -7.699999999999998401 ) ) ;
#29361=DIRECTION ( 'NONE',  ( 1.000000000000000000, -0.000000000000000000, -0.000000000000000000 ) ) ;
#29457=CARTESIAN_POINT ( 'NONE',  ( 186.5312500006828031, 9.429780353434619030E-16, -7.700000000000000178 ) ) ;
#29473=CARTESIAN_POINT ( 'NONE',  ( 185.0416666666666856, -4.445597072760122614, 7.699999999999998401 ) ) ;
#29716=CARTESIAN_POINT ( 'NONE',  ( 184.5052083336747444, -6.551208109652278289, 3.782341765624995134 ) ) ;
#29731=CIRCLE ( 'NONE', #102875, 4.000000000000000000 ) ;
#29736=DIRECTION ( 'NONE',  ( 1.000000000000000000, 0.000000000000000000, 0.000000000000000000 ) ) ;
#29917=CARTESIAN_POINT ( 'NONE',  ( 184.5000000000000000, 0.000000000000000000, 0.000000000000000000 ) ) ;
#29927=AXIS2_PLACEMENT_3D ( 'NONE', #38322, #40252, #110271 ) ;
#29941=CARTESIAN_POINT ( 'NONE',  ( 186.9062500006828316, -8.891194145520236347, -1.633285867636356693E-15 ) ) ;
#30319=FACE_OUTER_BOUND ( 'NONE', #58346, .T. ) ;
#30384=CARTESIAN_POINT ( 'NONE',  ( 184.8802083336747444, 4.367472073101515306, 7.564683531250000925 ) ) ;
#30642=ORIENTED_EDGE ( 'NONE', *, *, #114868, .T. ) ;
#30778=CARTESIAN_POINT ( 'NONE',  ( 184.1250000000000284, -8.891194145520236347, -1.633285867636356693E-15 ) ) ;
#30985=FACE_OUTER_BOUND ( 'NONE', #25353, .T. ) ;
#30995=EDGE_CURVE ( 'NONE', #97440, #70184, #107968, .T. ) ;
#31036=CARTESIAN_POINT ( 'NONE',  ( 185.1302083336747160, -4.367472073101514418, -7.564683531250002702 ) ) ;
#31184=CARTESIAN_POINT ( 'NONE',  ( 187.5000000000000000, -1.065442715258197248E-15, 8.699999999999999289 ) ) ;
#31236=CARTESIAN_POINT ( 'NONE',  ( 183.8645833340161175, -6.668395609140180369, 3.849999999999994760 ) ) ;
#31413=CARTESIAN_POINT ( 'NONE',  ( 184.2916666666666572, 4.445597072760120838, -7.699999999999998401 ) ) ;
#31562=CARTESIAN_POINT ( 'NONE',  ( 186.8385416670080872, 6.551208109652274736, 3.782341765625001351 ) ) ;
#31647=CARTESIAN_POINT ( 'NONE',  ( 184.5260416670080588, -6.551208109652273848, -3.782341765625003571 ) ) ;
#31654=CARTESIAN_POINT ( 'NONE',  ( 184.2135416670080588, 4.367472073101518859, -7.564683531249999149 ) ) ;
#31742=CIRCLE ( 'NONE', #125805, 5.200000000000000178 ) ;
#31814=CARTESIAN_POINT ( 'NONE',  ( 186.0000000000000000, 0.000000000000000000, 7.700000000000000178 ) ) ;
#31870=CARTESIAN_POINT ( 'NONE',  ( 187.0260416670080588, -6.551208109652273848, -3.782341765625003571 ) ) ;
#31884=ORIENTED_EDGE ( 'NONE', *, *, #12521, .F. ) ;
#32047=AXIS2_PLACEMENT_3D ( 'NONE', #58810, #29361, #69252 ) ;
#32066=CARTESIAN_POINT ( 'NONE',  ( 184.7916666666666856, 4.445597072760120838, -7.699999999999998401 ) ) ;
#32186=CARTESIAN_POINT ( 'NONE',  ( 184.4999999999999716, -7.210521358426481342, 2.491478058008155472 ) ) ;
#32478=VERTEX_POINT ( 'NONE', #62120 ) ;
#32482=CARTESIAN_POINT ( 'NONE',  ( 186.4427083336747160, -6.551208109652278289, 3.782341765624995134 ) ) ;
#32533=CARTESIAN_POINT ( 'NONE',  ( 185.4895833340161175, -4.445597072760115509, -7.700000000000001954 ) ) ;
#32635=( BOUNDED_CURVE ( )  B_SPLINE_CURVE ( 2, ( #19371, #80254, #69778, #70426, #50155, #99255, #101177 ),
 .UNSPECIFIED., .F., .F. ) 
 B_SPLINE_CURVE_WITH_KNOTS ( ( 3, 2, 2, 3 ),
 ( 0.2857142857142859760, 0.3095238095238098119, 0.3333333333333335924, 0.3571428571428574283 ),
 .UNSPECIFIED. ) 
 CURVE ( )  GEOMETRIC_REPRESENTATION_ITEM ( )  RATIONAL_B_SPLINE_CURVE ( ( 0.9999999999999984457, 0.8660254037844402619, 1.000000000000000000, 0.8660254037844387076, 1.000000000000000000, 0.8660254037844371533, 1.000000000000001554 ) ) 
 REPRESENTATION_ITEM ( '' )  );
#32867=CARTESIAN_POINT ( 'NONE',  ( 185.8802083336747444, 4.367472073101515306, 7.564683531250000925 ) ) ;
#32869=CARTESIAN_POINT ( 'NONE',  ( 187.3385416670080872, 6.551208109652274736, 3.782341765625001351 ) ) ;
#32968=EDGE_CURVE ( 'NONE', #50143, #70524, #10776, .T. ) ;
#33033=VECTOR ( 'NONE', #53964, 1000.000000000000000 ) ;
#33117=CARTESIAN_POINT ( 'NONE',  ( 186.3177083336747160, 4.367472073101515306, 7.564683531250000925 ) ) ;
#33173=CARTESIAN_POINT ( 'NONE',  ( 184.4479166673494603, -6.668395609140176816, -3.850000000000003642 ) ) ;
#33337=FACE_OUTER_BOUND ( 'NONE', #17161, .T. ) ;
#33386=( BOUNDED_CURVE ( )  B_SPLINE_CURVE ( 2, ( #73452, #24367, #113380, #54462, #55117, #103581, #123834 ),
 .UNSPECIFIED., .F., .F. ) 
 B_SPLINE_CURVE_WITH_KNOTS ( ( 3, 2, 2, 3 ),
 ( 0.1428571428571429880, 0.1666666666666668239, 0.1904761904761906322, 0.2142857142857144681 ),
 .UNSPECIFIED. ) 
 CURVE ( )  GEOMETRIC_REPRESENTATION_ITEM ( )  RATIONAL_B_SPLINE_CURVE ( ( 0.9999999999999992228, 0.8660254037844394848, 1.000000000000000000, 0.8660254037844387076, 1.000000000000000000, 0.8660254037844375974, 1.000000000000001110 ) ) 
 REPRESENTATION_ITEM ( '' )  );
#33505=CARTESIAN_POINT ( 'NONE',  ( 184.9218750003414016, 0.000000000000000000, 7.564683531250000925 ) ) ;
#33507=CARTESIAN_POINT ( 'NONE',  ( 186.3385416670080872, 6.551208109652274736, 3.782341765625001351 ) ) ;
#33647=DIRECTION ( 'NONE',  ( 0.000000000000000000, 0.000000000000000000, -1.000000000000000000 ) ) ;
#33737=CARTESIAN_POINT ( 'NONE',  ( 185.0677083336747160, -4.367472073101514418, -7.564683531250002702 ) ) ;
#33781=TOROIDAL_SURFACE ( 'NONE', #12828, 3.500000000000000000, 0.5000000000000000000 ) ;
#33793=CARTESIAN_POINT ( 'NONE',  ( 187.3177083336747444, 4.367472073101515306, 7.564683531250000925 ) ) ;
#33928=ADVANCED_FACE ( 'NONE', ( #107833 ), #18154, .T. ) ;
#33966=ORIENTED_EDGE ( 'NONE', *, *, #102227, .F. ) ;
#34058=CARTESIAN_POINT ( 'NONE',  ( 186.7812500006828031, 0.000000000000000000, 7.700000000000000178 ) ) ;
#34141=CARTESIAN_POINT ( 'NONE',  ( 186.5885416670080872, -6.551208109652273848, -3.782341765625003571 ) ) ;
#34143=CARTESIAN_POINT ( 'NONE',  ( 185.0468750003414300, -8.734944146203032389, -1.604583208406767949E-15 ) ) ;
#34205=ORIENTED_EDGE ( 'NONE', *, *, #62571, .T. ) ;
#34244=CARTESIAN_POINT ( 'NONE',  ( 184.4843750003414016, -8.734944146203032389, -1.604583208406768146E-15 ) ) ;
#34265=CARTESIAN_POINT ( 'NONE',  ( 187.5000000000000000, 0.000000000000000000, -5.200000000000000178 ) ) ;
#34350=EDGE_LOOP ( 'NONE', ( #39642, #20580, #124664, #96789 ) ) ;
#34402=ORIENTED_EDGE ( 'NONE', *, *, #85379, .F. ) ;
#34408=CARTESIAN_POINT ( 'NONE',  ( 184.6510416670080588, 4.367472073101518859, -7.564683531249999149 ) ) ;
#34457=CARTESIAN_POINT ( 'NONE',  ( 186.9427083336747160, -6.551208109652278289, 3.782341765624995134 ) ) ;
#34524=CARTESIAN_POINT ( 'NONE',  ( 184.4999999999999716, -4.098321783458930945, -6.521161088353083279 ) ) ;
#34527=ORIENTED_EDGE ( 'NONE', *, *, #125920, .T. ) ;
#34798=CARTESIAN_POINT ( 'NONE',  ( 185.9218750003414016, 0.000000000000000000, 7.564683531250000925 ) ) ;
#34800=CARTESIAN_POINT ( 'NONE',  ( 185.0052083336747444, -6.551208109652278289, 3.782341765624995134 ) ) ;
#34836=CARTESIAN_POINT ( 'NONE',  ( 187.3593750003414016, 0.000000000000000000, 7.564683531250000925 ) ) ;
#34914=EDGE_CURVE ( 'NONE', #50143, #8279, #105279, .T. ) ;
#34917=VERTEX_POINT ( 'NONE', #56792 ) ;
#35049=CARTESIAN_POINT ( 'NONE',  ( 184.3177083336747160, 4.367472073101515306, 7.564683531250000925 ) ) ;
#35105=CARTESIAN_POINT ( 'NONE',  ( 185.9427083336747160, -6.551208109652278289, 3.782341765624995134 ) ) ;
#35369=EDGE_CURVE ( 'NONE', #99741, #99122, #53125, .T. ) ;
#35432=CARTESIAN_POINT ( 'NONE',  ( 186.3802083336747444, 4.367472073101515306, 7.564683531250000925 ) ) ;
#35436=CARTESIAN_POINT ( 'NONE',  ( 185.9218750003414016, 0.000000000000000000, 7.564683531250000925 ) ) ;
#35447=CARTESIAN_POINT ( 'NONE',  ( 187.2500000000000000, 9.429780353434619030E-16, -7.700000000000000178 ) ) ;
#35466=CARTESIAN_POINT ( 'NONE',  ( 187.2343750003414016, 8.734944146203032389, 5.348610694689227483E-16 ) ) ;
#35516=CARTESIAN_POINT ( 'NONE',  ( 184.7500000000000000, 9.429780353434619030E-16, -7.700000000000000178 ) ) ;
#35519=VERTEX_POINT ( 'NONE', #107039 ) ;
#35561=EDGE_LOOP ( 'NONE', ( #47138, #34527, #40650, #100260, #53877, #98163, #120185, #97684, #124096, #66708, #94191, #92556, #10611, #36738, #126128 ) ) ;
#35650=CARTESIAN_POINT ( 'NONE',  ( 187.4218750003414016, 0.000000000000000000, 7.564683531250000925 ) ) ;
#35678=CARTESIAN_POINT ( 'NONE',  ( 187.3802083336747444, 4.367472073101515306, 7.564683531250000925 ) ) ;
#35731=CARTESIAN_POINT ( 'NONE',  ( 184.7343750003414016, 8.734944146203032389, 5.348610694689227483E-16 ) ) ;
#35751=CARTESIAN_POINT ( 'NONE',  ( 184.5000000000000000, 0.000000000000000000, 0.000000000000000000 ) ) ;
#35912=DIRECTION ( 'NONE',  ( 1.000000000000000000, -0.000000000000000000, -0.000000000000000000 ) ) ;
#36068=CARTESIAN_POINT ( 'NONE',  ( 185.8750000000000000, 8.891194145520236347, 5.444286225454521982E-16 ) ) ;
#36070=CARTESIAN_POINT ( 'NONE',  ( 184.5000000000000000, -6.267304879582558996, 4.236192450104883100 ) ) ;
#36106=CARTESIAN_POINT ( 'NONE',  ( 186.3177083336747160, 4.367472073101515306, 7.564683531250000925 ) ) ;
#36167=DIRECTION ( 'NONE',  ( 0.000000000000000000, 0.000000000000000000, -1.000000000000000000 ) ) ;
#36291=PRODUCT_DEFINITION_CONTEXT ( 'detailed design', #4514, 'design' ) ;
#36341=CARTESIAN_POINT ( 'NONE',  ( 186.9218750003414016, 0.000000000000000000, 7.564683531250000925 ) ) ;
#36380=VERTEX_POINT ( 'NONE', #6572 ) ;
#36393=CARTESIAN_POINT ( 'NONE',  ( 185.9843750003414016, -8.734944146203032389, -1.604583208406768146E-15 ) ) ;
#36476=ORIENTED_EDGE ( 'NONE', *, *, #121353, .F. ) ;
#36621=ORIENTED_EDGE ( 'NONE', *, *, #8218, .T. ) ;
#36647=FACE_OUTER_BOUND ( 'NONE', #24847, .T. ) ;
#36649=CARTESIAN_POINT ( 'NONE',  ( 185.0000000000000000, 0.000000000000000000, 7.700000000000000178 ) ) ;
#36662=VERTEX_POINT ( 'NONE', #56029 ) ;
#36698=CARTESIAN_POINT ( 'NONE',  ( 186.2812500006828031, 0.000000000000000000, 7.700000000000000178 ) ) ;
#36726=CARTESIAN_POINT ( 'NONE',  ( 186.7916666666666572, 4.445597072760120838, -7.699999999999998401 ) ) ;
#36729=CARTESIAN_POINT ( 'NONE',  ( 185.2135416670080588, 4.367472073101518859, -7.564683531249999149 ) ) ;
#36738=ORIENTED_EDGE ( 'NONE', *, *, #32968, .T. ) ;
#36760=CARTESIAN_POINT ( 'NONE',  ( 187.0260416670080588, -6.551208109652273848, -3.782341765625003571 ) ) ;
#36846=FACE_OUTER_BOUND ( 'NONE', #21386, .T. ) ;
#36854=ORIENTED_EDGE ( 'NONE', *, *, #49126, .T. ) ;
#36969=CARTESIAN_POINT ( 'NONE',  ( 185.6718750003414016, 9.264065473108010111E-16, -7.564683531250000925 ) ) ;
#37086=AXIS2_PLACEMENT_3D ( 'NONE', #102981, #22519, #62436 ) ;
#37228=VECTOR ( 'NONE', #83687, 1000.000000000000000 ) ;
#37304=( GEOMETRIC_REPRESENTATION_CONTEXT ( 3 ) GLOBAL_UNCERTAINTY_ASSIGNED_CONTEXT ( ( #99057 ) ) GLOBAL_UNIT_ASSIGNED_CONTEXT ( ( #67478, #9879, #49821 ) ) REPRESENTATION_CONTEXT ( 'NONE', 'WORKASPACE' ) );
#37372=CARTESIAN_POINT ( 'NONE',  ( 186.9583333333333428, 4.445597072760117285, 7.699999999999999289 ) ) ;
#37400=CARTESIAN_POINT ( 'NONE',  ( 184.7760416670080588, 6.551208109652274736, 3.782341765625001351 ) ) ;
#37619=CARTESIAN_POINT ( 'NONE',  ( 186.5468750003414300, -8.734944146203032389, -1.604583208406768146E-15 ) ) ;
#37698=CARTESIAN_POINT ( 'NONE',  ( 184.4999999999999716, -4.613861370277991369, 6.083321009326518869 ) ) ;
#37893=DIRECTION ( 'NONE',  ( 1.000000000000000000, -0.000000000000000000, -0.000000000000000000 ) ) ;
#37909=DIRECTION ( 'NONE',  ( 0.000000000000000000, 0.000000000000000000, -1.000000000000000000 ) ) ;
#37996=CARTESIAN_POINT ( 'NONE',  ( 187.0416666666666288, -4.445597072760122614, 7.699999999999998401 ) ) ;
#38029=CARTESIAN_POINT ( 'NONE',  ( 185.7343750003414016, 8.734944146203032389, 5.348610694689227483E-16 ) ) ;
#38053=FILL_AREA_STYLE ('',( #79277 ) ) ;
#38138=AXIS2_PLACEMENT_3D ( 'NONE', #28772, #88971, #109907 ) ;
#38262=CARTESIAN_POINT ( 'NONE',  ( 184.0677083336747160, -4.367472073101514418, -7.564683531250002702 ) ) ;
#38319=FACE_OUTER_BOUND ( 'NONE', #118677, .T. ) ;
#38322=CARTESIAN_POINT ( 'NONE',  ( 184.5000000000000000, 0.000000000000000000, 0.000000000000000000 ) ) ;
#38452=EDGE_CURVE ( 'NONE', #55284, #70524, #44080, .T. ) ;
#38572=DIRECTION ( 'NONE',  ( 0.000000000000000000, 0.000000000000000000, -1.000000000000000000 ) ) ;
#38635=EDGE_CURVE ( 'NONE', #36662, #53828, #82700, .T. ) ;
#38670=CARTESIAN_POINT ( 'NONE',  ( 185.7083333333333428, -4.445597072760115509, -7.700000000000001954 ) ) ;
#38727=SHAPE_REPRESENTATION_RELATIONSHIP ( 'NONE' , 'NONE' ,  #18450, #25840 ) ;
#39012=ADVANCED_FACE ( 'NONE', ( #30319 ), #29023, .T. ) ;
#39142=CARTESIAN_POINT ( 'NONE',  ( 186.2395833340161460, 4.445597072760117285, 7.699999999999999289 ) ) ;
#39170=VERTEX_POINT ( 'NONE', #123815 ) ;
#39212=CARTESIAN_POINT ( 'NONE',  ( 195.0000000000000000, 0.000000000000000000, 0.000000000000000000 ) ) ;
#39323=CARTESIAN_POINT ( 'NONE',  ( 184.5833333333333144, -6.668395609140180369, 3.849999999999994760 ) ) ;
#39349=CARTESIAN_POINT ( 'NONE',  ( 185.4843750003414016, -8.734944146203032389, -1.604583208406767949E-15 ) ) ;
#39473=CARTESIAN_POINT ( 'NONE',  ( 185.6666666666666856, -6.668395609140176816, -3.850000000000003642 ) ) ;
#39495=ORIENTED_EDGE ( 'NONE', *, *, #102895, .F. ) ;
#39529=EDGE_CURVE ( 'NONE', #41594, #32478, #87180, .T. ) ;
#39540=ORIENTED_EDGE ( 'NONE', *, *, #80486, .F. ) ;
#39642=ORIENTED_EDGE ( 'NONE', *, *, #27677, .T. ) ;
#39724=CARTESIAN_POINT ( 'NONE',  ( 187.3593750003414016, 0.000000000000000000, 7.564683531250000925 ) ) ;
#39777=CARTESIAN_POINT ( 'NONE',  ( 187.1145833340161175, 6.668395609140177704, -3.849999999999998312 ) ) ;
#39937=DIRECTION ( 'NONE',  ( 1.000000000000000000, 0.000000000000000000, 0.000000000000000000 ) ) ;
#39988=EDGE_CURVE ( 'NONE', #28707, #58259, #91863, .T. ) ;
#40093=EDGE_LOOP ( 'NONE', ( #3819, #30642, #47044, #26753 ) ) ;
#40190=CARTESIAN_POINT ( 'NONE',  ( 183.9635416670080872, -4.367472073101519747, 7.564683531249999149 ) ) ;
#40198=CIRCLE ( 'NONE', #113335, 5.000000000000000000 ) ;
#40252=DIRECTION ( 'NONE',  ( 1.000000000000000000, -0.000000000000000000, -0.000000000000000000 ) ) ;
#40311=EDGE_CURVE ( 'NONE', #36380, #54095, #117824, .T. ) ;
#40352=CARTESIAN_POINT ( 'NONE',  ( 187.1510416670080303, 4.367472073101518859, -7.564683531249999149 ) ) ;
#40390=DIRECTION ( 'NONE',  ( 1.000000000000000000, -0.000000000000000000, -0.000000000000000000 ) ) ;
#40635=EDGE_CURVE ( 'NONE', #22601, #44517, #10429, .T. ) ;
#40650=ORIENTED_EDGE ( 'NONE', *, *, #73518, .T. ) ;
#40768=DIRECTION ( 'NONE',  ( 0.000000000000000000, 0.000000000000000000, 1.000000000000000000 ) ) ;
#40856=CARTESIAN_POINT ( 'NONE',  ( 185.0052083336747444, -6.551208109652278289, 3.782341765624995134 ) ) ;
#40884=ADVANCED_FACE ( 'NONE', ( #54952 ), #45795, .F. ) ;
#40909=ORIENTED_EDGE ( 'NONE', *, *, #40635, .T. ) ;
#41000=EDGE_CURVE ( 'NONE', #97220, #28707, #115134, .T. ) ;
#41006=ORIENTED_EDGE ( 'NONE', *, *, #126863, .F. ) ;
#41030=( BOUNDED_CURVE ( )  B_SPLINE_CURVE ( 2, ( #115397, #44774, #106258, #16564, #96419, #45416, #65018 ),
 .UNSPECIFIED., .F., .F. ) 
 B_SPLINE_CURVE_WITH_KNOTS ( ( 3, 2, 2, 3 ),
 ( 0.5714285714285719520, 0.5952380952380957879, 0.6190476190476195129, 0.6428571428571433488 ),
 .UNSPECIFIED. ) 
 CURVE ( )  GEOMETRIC_REPRESENTATION_ITEM ( )  RATIONAL_B_SPLINE_CURVE ( ( 0.9999999999999968914, 0.8660254037844418162, 1.000000000000000000, 0.8660254037844387076, 1.000000000000000000, 0.8660254037844361541, 1.000000000000002442 ) ) 
 REPRESENTATION_ITEM ( '' )  );
#41067=CARTESIAN_POINT ( 'NONE',  ( 185.0312500006828031, 9.429780353434619030E-16, -7.700000000000000178 ) ) ;
#41241=CARTESIAN_POINT ( 'NONE',  ( 184.4166666666666856, 6.668395609140176816, 3.850000000000000977 ) ) ;
#41261=( BOUNDED_CURVE ( )  B_SPLINE_CURVE ( 2, ( #36698, #107347, #97525, #7852, #5905, #45868, #116520 ),
 .UNSPECIFIED., .F., .F. ) 
 B_SPLINE_CURVE_WITH_KNOTS ( ( 3, 2, 2, 3 ),
 ( 0.2857142857142859760, 0.3095238095238098119, 0.3333333333333335924, 0.3571428571428574283 ),
 .UNSPECIFIED. ) 
 CURVE ( )  GEOMETRIC_REPRESENTATION_ITEM ( )  RATIONAL_B_SPLINE_CURVE ( ( 0.9999999999999984457, 0.8660254037844402619, 1.000000000000000000, 0.8660254037844387076, 1.000000000000000000, 0.8660254037844371533, 1.000000000000001554 ) ) 
 REPRESENTATION_ITEM ( '' )  );
#41291=DIRECTION ( 'NONE',  ( 1.000000000000000000, 0.000000000000000000, 0.000000000000000000 ) ) ;
#41346=DIRECTION ( 'NONE',  ( 0.000000000000000000, -1.000000000000000000, 0.000000000000000000 ) ) ;
#41501=CARTESIAN_POINT ( 'NONE',  ( 184.5468750003414300, -8.734944146203032389, -1.604583208406768146E-15 ) ) ;
#41594=VERTEX_POINT ( 'NONE', #82080 ) ;
#41693=ORIENTED_EDGE ( 'NONE', *, *, #80341, .T. ) ;
#41695=ORIENTED_EDGE ( 'NONE', *, *, #40635, .F. ) ;
#41703=CARTESIAN_POINT ( 'NONE',  ( 187.1093750003414016, 9.264065473108010111E-16, -7.564683531250000925 ) ) ;
#41764=DIRECTION ( 'NONE',  ( -1.000000000000000000, -0.000000000000000000, -0.000000000000000000 ) ) ;
#41805=EDGE_CURVE ( 'NONE', #91613, #36380, #127038, .T. ) ;
#41818=LINE ( 'NONE', #81709, #63026 ) ;
#41883=CARTESIAN_POINT ( 'NONE',  ( 184.7083333333333144, -4.445597072760115509, -7.700000000000001954 ) ) ;
#42114=CIRCLE ( 'NONE', #115224, 5.000000000000000000 ) ;
#42214=CARTESIAN_POINT ( 'NONE',  ( 185.2916666666666572, 4.445597072760072876, -7.700000000000080114 ) ) ;
#42280=EDGE_CURVE ( 'NONE', #53828, #36380, #16377, .T. ) ;
#42320=DIRECTION ( 'NONE',  ( 0.000000000000000000, 0.000000000000000000, -1.000000000000000000 ) ) ;
#42333=CARTESIAN_POINT ( 'NONE',  ( 184.1979166673494603, 6.668395609140176816, 3.850000000000000977 ) ) ;
#42481=DIRECTION ( 'NONE',  ( 1.000000000000000000, -0.000000000000000000, -0.000000000000000000 ) ) ;
#42521=ORIENTED_EDGE ( 'NONE', *, *, #64751, .F. ) ;
#42567=VECTOR ( 'NONE', #28970, 1000.000000000000000 ) ;
#42691=CARTESIAN_POINT ( 'NONE',  ( 187.2552083336747444, 6.551208109652275624, -3.782341765624998686 ) ) ;
#42694=CARTESIAN_POINT ( 'NONE',  ( 186.9218750003414016, 0.000000000000000000, 7.564683531250000925 ) ) ;
#42768=CARTESIAN_POINT ( 'NONE',  ( 187.5000000000000000, 0.000000000000000000, -7.699999999999999289 ) ) ;
#42774=ORIENTED_EDGE ( 'NONE', *, *, #84262, .T. ) ;
#42874=CARTESIAN_POINT ( 'NONE',  ( 184.5000000000000000, 0.000000000000000000, 0.000000000000000000 ) ) ;
#42947=CARTESIAN_POINT ( 'NONE',  ( 185.8593750003413732, 0.000000000000000000, 7.564683531250000925 ) ) ;
#43006=CARTESIAN_POINT ( 'NONE',  ( 185.6562500006828316, 8.891194145520236347, 5.444286225454521982E-16 ) ) ;
#43196=ORIENTED_EDGE ( 'NONE', *, *, #23726, .T. ) ;
#43278=DIRECTION ( 'NONE',  ( 0.000000000000000000, 0.000000000000000000, -1.000000000000000000 ) ) ;
#43300=ORIENTED_EDGE ( 'NONE', *, *, #69291, .F. ) ;
#43325=CARTESIAN_POINT ( 'NONE',  ( 184.7135416670080872, 4.367472073101518859, -7.564683531249999149 ) ) ;
#43327=CARTESIAN_POINT ( 'NONE',  ( 186.3802083336747444, 4.367472073101515306, 7.564683531250000925 ) ) ;
#43474=DIRECTION ( 'NONE',  ( 0.000000000000000000, 1.000000000000000000, -1.224646799147353207E-16 ) ) ;
#43580=CARTESIAN_POINT ( 'NONE',  ( 185.1510416670080872, 4.367472073101518859, -7.564683531249999149 ) ) ;
#43584=CARTESIAN_POINT ( 'NONE',  ( 186.0000000000000000, 0.000000000000000000, 7.700000000000000178 ) ) ;
#43620=ORIENTED_EDGE ( 'NONE', *, *, #2762, .T. ) ;
#43636=CARTESIAN_POINT ( 'NONE',  ( 185.5729166673494319, 4.445597072760120838, -7.699999999999998401 ) ) ;
#43690=AXIS2_PLACEMENT_3D ( 'NONE', #125547, #26076, #76464 ) ;
#43798=CARTESIAN_POINT ( 'NONE',  ( 187.4609375001707008, 0.000000000000000000, 7.632341765625000107 ) ) ;
#43886=CARTESIAN_POINT ( 'NONE',  ( 186.5000000000000000, 0.000000000000000000, 7.700000000000000178 ) ) ;
#43931=ORIENTED_EDGE ( 'NONE', *, *, #27415, .T. ) ;
#43938=CARTESIAN_POINT ( 'NONE',  ( 194.5000000000000000, 0.000000000000000000, 0.000000000000000000 ) ) ;
#43961=CARTESIAN_POINT ( 'NONE',  ( 185.7968750003414300, 8.734944146203032389, 5.348610694689227483E-16 ) ) ;
#44080=B_SPLINE_CURVE_WITH_KNOTS ( 'NONE', 3,
 ( #47520, #87423, #127368, #37698, #77599, #67789, #97890, #91300, #110926, #109660, #59935, #71026 ),
 .UNSPECIFIED., .F., .F.,
 ( 4, 2, 2, 2, 2, 4 ),
 ( 0.000000000000000000, 0.001866281188413360234, 0.003732562376826720468, 0.005598843565240080485, 0.006531984159446760710, 0.007465124753653440935 ),
 .UNSPECIFIED. ) ;
#44172=DIRECTION ( 'NONE',  ( 1.000000000000000000, 0.000000000000000000, 0.000000000000000000 ) ) ;
#44192=CARTESIAN_POINT ( 'NONE',  ( 185.9427083336747160, -6.551208109652278289, 3.782341765624995134 ) ) ;
#44198=VECTOR ( 'NONE', #85389, 1000.000000000000000 ) ;
#44217=EDGE_CURVE ( 'NONE', #86499, #58259, #45593, .T. ) ;
#44248=CARTESIAN_POINT ( 'NONE',  ( 186.5677083336747160, -4.367472073101514418, -7.564683531250002702 ) ) ;
#44286=ORIENTED_EDGE ( 'NONE', *, *, #112824, .T. ) ;
#44402=CARTESIAN_POINT ( 'NONE',  ( 187.5000000000000000, 0.000000000000000000, -8.699999999999999289 ) ) ;
#44455=CARTESIAN_POINT ( 'NONE',  ( 184.5000000000000000, -7.430520870378829024, -1.418378131116527108 ) ) ;
#44517=VERTEX_POINT ( 'NONE', #21772 ) ;
#44599=CARTESIAN_POINT ( 'NONE',  ( 186.6302083336747160, -4.367472073101514418, -7.564683531250002702 ) ) ;
#44748=CARTESIAN_POINT ( 'NONE',  ( 185.5729166673494603, 4.445597072760072876, -7.700000000000080114 ) ) ;
#44774=CARTESIAN_POINT ( 'NONE',  ( 185.2395833340161460, 4.445597072760175905, 7.699999999999896261 ) ) ;
#44861=CARTESIAN_POINT ( 'NONE',  ( 184.4427083336747160, -6.551208109652278289, 3.782341765624995134 ) ) ;
#44915=CARTESIAN_POINT ( 'NONE',  ( 186.7343750003414300, 8.734944146203032389, 5.348610694689227483E-16 ) ) ;
#44981=CARTESIAN_POINT ( 'NONE',  ( 184.4999999999999716, -7.141846329728243958, -2.638575396834020648 ) ) ;
#44988=ORIENTED_EDGE ( 'NONE', *, *, #102227, .T. ) ;
#45060=ORIENTED_EDGE ( 'NONE', *, *, #35369, .F. ) ;
#45202=LINE ( 'NONE', #83816, #88483 ) ;
#45224=CYLINDRICAL_SURFACE ( 'NONE', #54323, 5.000000000000000000 ) ;
#45247=CARTESIAN_POINT ( 'NONE',  ( 186.0052083336747444, -6.551208109652278289, 3.782341765624995134 ) ) ;
#45287=CARTESIAN_POINT ( 'NONE',  ( 186.6093750003414016, 9.264065473108010111E-16, -7.564683531250000925 ) ) ;
#45339=CARTESIAN_POINT ( 'NONE',  ( 185.9895833340161175, -4.445597072760145707, -7.699999999999951328 ) ) ;
#45392=CARTESIAN_POINT ( 'NONE',  ( 185.7812500006828031, 0.000000000000000000, 7.700000000000000178 ) ) ;
#45416=CARTESIAN_POINT ( 'NONE',  ( 185.0729166673495172, 4.445597072760072876, -7.700000000000080114 ) ) ;
#45484=CARTESIAN_POINT ( 'NONE',  ( 187.3906250003414016, 0.000000000000000000, 7.700000000000000178 ) ) ;
#45510=CARTESIAN_POINT ( 'NONE',  ( 184.8593750003413732, 0.000000000000000000, 7.564683531250000925 ) ) ;
#45564=CARTESIAN_POINT ( 'NONE',  ( 184.9843750003414016, -8.734944146203032389, -1.604583208406768146E-15 ) ) ;
#45593=LINE ( 'NONE', #95969, #3320 ) ;
#45795=PLANE ( 'NONE',  #128082 ) ;
#45868=CARTESIAN_POINT ( 'NONE',  ( 186.0729166673494603, 4.445597072760091528, -7.700000000000049916 ) ) ;
#45892=CARTESIAN_POINT ( 'NONE',  ( 184.8385416670080872, 6.551208109652274736, 3.782341765625001351 ) ) ;
#45895=CARTESIAN_POINT ( 'NONE',  ( 185.4635416670080872, -4.367472073101520635, 7.564683531249999149 ) ) ;
#45933=CARTESIAN_POINT ( 'NONE',  ( 186.5677083336747160, -4.367472073101514418, -7.564683531250002702 ) ) ;
#45988=CARTESIAN_POINT ( 'NONE',  ( 184.5000000000000000, 0.000000000000000000, 0.000000000000000000 ) ) ;
#46124=ADVANCED_FACE ( 'NONE', ( #3198 ), #103324, .T. ) ;
#46134=CARTESIAN_POINT ( 'NONE',  ( 186.6718750003414016, 9.264065473108010111E-16, -7.564683531250000925 ) ) ;
#46190=CARTESIAN_POINT ( 'NONE',  ( 186.6927083336747160, 6.551208109652275624, -3.782341765624998686 ) ) ;
#46466=ADVANCED_FACE ( 'NONE', ( #90097 ), #50843, .F. ) ;
#46515=CARTESIAN_POINT ( 'NONE',  ( 186.0416666666666856, -4.445597072760122614, 7.699999999999998401 ) ) ;
#46517=CARTESIAN_POINT ( 'NONE',  ( 186.1718750003414016, 9.264065473108010111E-16, -7.564683531250000925 ) ) ;
#46548=CARTESIAN_POINT ( 'NONE',  ( 186.4427083336747160, -6.551208109652278289, 3.782341765624995134 ) ) ;
#46562=AXIS2_PLACEMENT_3D ( 'NONE', #84829, #56640, #104470 ) ;
#46791=CARTESIAN_POINT ( 'NONE',  ( 185.2968750003414300, 8.734944146203032389, 5.348610694689227483E-16 ) ) ;
#46842=EDGE_LOOP ( 'NONE', ( #86111, #86616, #1422, #52560 ) ) ;
#47034=ADVANCED_FACE ( 'NONE', ( #55027 ), #45224, .F. ) ;
#47044=ORIENTED_EDGE ( 'NONE', *, *, #41805, .T. ) ;
#47088=DIRECTION ( 'NONE',  ( 1.000000000000000000, 0.000000000000000000, 0.000000000000000000 ) ) ;
#47108=CARTESIAN_POINT ( 'NONE',  ( 185.1666666666666856, -6.668395609140176816, -3.850000000000003642 ) ) ;
#47116=ORIENTED_EDGE ( 'NONE', *, *, #3429, .F. ) ;
#47138=ORIENTED_EDGE ( 'NONE', *, *, #25458, .F. ) ;
#47185=CARTESIAN_POINT ( 'NONE',  ( 186.6250000000000284, -8.891194145520236347, -1.633285867636356693E-15 ) ) ;
#47187=CARTESIAN_POINT ( 'NONE',  ( 185.3802083336747444, 4.367472073101515306, 7.564683531250000925 ) ) ;
#47215=CARTESIAN_POINT ( 'NONE',  ( 184.7343750003414016, 8.734944146203032389, 5.348610694689227483E-16 ) ) ;
#47237=PRESENTATION_STYLE_ASSIGNMENT (( #107432 ) ) ;
#47435=CARTESIAN_POINT ( 'NONE',  ( 187.0885416670080872, -6.551208109652273848, -3.782341765625003571 ) ) ;
#47520=CARTESIAN_POINT ( 'NONE',  ( 184.5000000000000000, -6.267304879582558996, 4.236192450104883100 ) ) ;
#47541=CARTESIAN_POINT ( 'NONE',  ( 194.5000000000000000, 0.000000000000000000, -5.000000000000000000 ) ) ;
#47594=EDGE_CURVE ( 'NONE', #108189, #52320, #100103, .T. ) ;
#47629=DIRECTION ( 'NONE',  ( 0.000000000000000000, 0.000000000000000000, -1.000000000000000000 ) ) ;
#47702=EDGE_LOOP ( 'NONE', ( #47116, #73659, #82972, #41006 ) ) ;
#47836=CARTESIAN_POINT ( 'NONE',  ( 186.2083333333333144, -4.445597072760115509, -7.700000000000001954 ) ) ;
#48082=CARTESIAN_POINT ( 'NONE',  ( 185.5052083336747444, -6.551208109652278289, 3.782341765624995134 ) ) ;
#48164=ORIENTED_EDGE ( 'NONE', *, *, #16235, .F. ) ;
#48239=DIRECTION ( 'NONE',  ( -1.000000000000000000, 0.000000000000000000, 0.000000000000000000 ) ) ;
#48348=CARTESIAN_POINT ( 'NONE',  ( 194.5000000000000000, 6.123233995736766282E-16, 5.000000000000000000 ) ) ;
#48372=ADVANCED_FACE ( 'NONE', ( #71630 ), #3536, .T. ) ;
#48463=CARTESIAN_POINT ( 'NONE',  ( 185.7916666666666572, 4.445597072760120838, -7.699999999999998401 ) ) ;
#48480=DIRECTION ( 'NONE',  ( 0.000000000000000000, 0.000000000000000000, -1.000000000000000000 ) ) ;
#48538=DIRECTION ( 'NONE',  ( 0.000000000000000000, 0.000000000000000000, -1.000000000000000000 ) ) ;
#48602=LINE ( 'NONE', #128467, #42567 ) ;
#48727=CARTESIAN_POINT ( 'NONE',  ( 184.7135416670080872, 4.367472073101518859, -7.564683531249999149 ) ) ;
#48941=CARTESIAN_POINT ( 'NONE',  ( 186.4895833340161175, -4.445597072760115509, -7.700000000000001954 ) ) ;
#49047=CARTESIAN_POINT ( 'NONE',  ( 184.5312500006828031, 9.429780353434619030E-16, -7.700000000000000178 ) ) ;
#49095=EDGE_LOOP ( 'NONE', ( #124256, #56400, #43620, #67947 ) ) ;
#49126=EDGE_CURVE ( 'NONE', #109569, #17430, #125041, .T. ) ;
#49131=CARTESIAN_POINT ( 'NONE',  ( 184.2135416670080588, 4.367472073101518859, -7.564683531249999149 ) ) ;
#49164=CARTESIAN_POINT ( 'NONE',  ( 184.5677083336747444, -4.367472073101514418, -7.564683531250002702 ) ) ;
#49216=ORIENTED_EDGE ( 'NONE', *, *, #52059, .F. ) ;
#49363=AXIS2_PLACEMENT_3D ( 'NONE', #23115, #74159, #83957 ) ;
#49380=CARTESIAN_POINT ( 'NONE',  ( 185.0885416670080872, -6.551208109652273848, -3.782341765625003571 ) ) ;
#49386=CARTESIAN_POINT ( 'NONE',  ( 187.5000000000000000, 0.000000000000000000, 0.000000000000000000 ) ) ;
#49569=CARTESIAN_POINT ( 'NONE',  ( 184.5416666666666572, -4.445597072760039126, 7.700000000000142286 ) ) ;
#49591=CARTESIAN_POINT ( 'NONE',  ( 187.1562500006828316, 8.891194145520236347, 5.444286225454521982E-16 ) ) ;
#49640=CARTESIAN_POINT ( 'NONE',  ( 186.6562500006828031, 8.891194145520236347, 5.444286225454521982E-16 ) ) ;
#49668=AXIS2_PLACEMENT_3D ( 'NONE', #54336, #55624, #64791 ) ;
#49760=CARTESIAN_POINT ( 'NONE',  ( 184.5000000000000000, 0.000000000000000000, -7.699999999999999289 ) ) ;
#49777=CARTESIAN_POINT ( 'NONE',  ( 184.3333333333333144, 6.668395609140177704, -3.849999999999998312 ) ) ;
#49821=( NAMED_UNIT ( * ) SI_UNIT ( $, .STERADIAN. ) SOLID_ANGLE_UNIT ( ) );
#49959=VECTOR ( 'NONE', #125481, 1000.000000000000000 ) ;
#50005=EDGE_LOOP ( 'NONE', ( #22442, #79368, #2130, #16439 ) ) ;
#50029=CARTESIAN_POINT ( 'NONE',  ( 184.2968750003414300, 8.734944146203032389, 5.348610694689227483E-16 ) ) ;
#50143=VERTEX_POINT ( 'NONE', #23693 ) ;
#50155=CARTESIAN_POINT ( 'NONE',  ( 186.3333333333333144, 6.668395609140177704, -3.849999999999998312 ) ) ;
#50232=CARTESIAN_POINT ( 'NONE',  ( 187.0729166673494319, 4.445597072760120838, -7.699999999999998401 ) ) ;
#50457=CARTESIAN_POINT ( 'NONE',  ( 186.9479166673494603, -6.668395609140176816, -3.850000000000003642 ) ) ;
#50843=CYLINDRICAL_SURFACE ( 'NONE', #123196, 5.200000000000000178 ) ;
#50847=AXIS2_PLACEMENT_3D ( 'NONE', #49386, #89289, #80117 ) ;
#50865=CARTESIAN_POINT ( 'NONE',  ( 185.9062500006828316, -8.891194145520236347, -1.633285867636356693E-15 ) ) ;
#50971=CARTESIAN_POINT ( 'NONE',  ( 194.5000000000000000, 6.123233995736766282E-16, 5.000000000000000000 ) ) ;
#51060=CARTESIAN_POINT ( 'NONE',  ( 184.1666666666666856, -6.668395609140176816, -3.850000000000003642 ) ) ;
#51062=VECTOR ( 'NONE', #620, 1000.000000000000000 ) ;
#51135=CIRCLE ( 'NONE', #86610, 8.040022453829767102 ) ;
#51179=EDGE_CURVE ( 'NONE', #67593, #41594, #100034, .T. ) ;
#51315=CARTESIAN_POINT ( 'NONE',  ( 184.6718750003414016, 9.264065473108010111E-16, -7.564683531250000925 ) ) ;
#51497=CIRCLE ( 'NONE', #49363, 8.040022453829767102 ) ;
#51515=CARTESIAN_POINT ( 'NONE',  ( 183.8229166673494888, -4.445597072760122614, 7.699999999999998401 ) ) ;
#51697=CARTESIAN_POINT ( 'NONE',  ( 185.2083333333333144, -4.445597072760115509, -7.700000000000001954 ) ) ;
#51809=EDGE_LOOP ( 'NONE', ( #31884, #71690, #11135, #94131 ) ) ;
#51852=CARTESIAN_POINT ( 'NONE',  ( 187.1718750003414016, 9.264065473108010111E-16, -7.564683531250000925 ) ) ;
#51922=CARTESIAN_POINT ( 'NONE',  ( 194.5000000000000000, 0.000000000000000000, -4.000000000000000000 ) ) ;
#51939=CARTESIAN_POINT ( 'NONE',  ( 183.9010416670080588, -4.367472073101519747, 7.564683531249999149 ) ) ;
#52059=EDGE_CURVE ( 'NONE', #108189, #28707, #76225, .T. ) ;
#52063=VERTEX_POINT ( 'NONE', #35650 ) ;
#52152=CARTESIAN_POINT ( 'NONE',  ( 184.4895833340161460, -4.445597072760115509, -7.700000000000001954 ) ) ;
#52217=CARTESIAN_POINT ( 'NONE',  ( 184.4999999999999432, -7.324530227482785705, -2.036292321216437884 ) ) ;
#52320=VERTEX_POINT ( 'NONE', #42768 ) ;
#52495=ORIENTED_EDGE ( 'NONE', *, *, #68206, .T. ) ;
#52560=ORIENTED_EDGE ( 'NONE', *, *, #2762, .F. ) ;
#52566=CARTESIAN_POINT ( 'NONE',  ( 183.8593750003413732, 0.000000000000000000, 7.564683531250000925 ) ) ;
#52602=EDGE_CURVE ( 'NONE', #79758, #67593, #40198, .T. ) ;
#52730=CARTESIAN_POINT ( 'NONE',  ( 186.1093750003413732, 9.264065473108010111E-16, -7.564683531250000925 ) ) ;
#52788=CARTESIAN_POINT ( 'NONE',  ( 184.3229166673494603, -4.445597072760122614, 7.699999999999998401 ) ) ;
#52856=CARTESIAN_POINT ( 'NONE',  ( 184.4999999999999716, -6.306458657965935188, -4.321730308584150748 ) ) ;
#53002=FACE_OUTER_BOUND ( 'NONE', #12681, .T. ) ;
#53104=EDGE_CURVE ( 'NONE', #53828, #121663, #91083, .T. ) ;
#53125=CIRCLE ( 'NONE', #46562, 4.000000000000000000 ) ;
#53134=CARTESIAN_POINT ( 'NONE',  ( 185.4218750003414016, 0.000000000000000000, 7.564683531250000925 ) ) ;
#53136=CARTESIAN_POINT ( 'NONE',  ( 186.7968750003414300, 8.734944146203032389, 5.348610694689227483E-16 ) ) ;
#53224=CARTESIAN_POINT ( 'NONE',  ( 184.8750000000000000, 8.891194145520236347, 5.444286225454521982E-16 ) ) ;
#53261=ORIENTED_EDGE ( 'NONE', *, *, #32968, .F. ) ;
#53369=VECTOR ( 'NONE', #1617, 1000.000000000000000 ) ;
#53388=CARTESIAN_POINT ( 'NONE',  ( 185.5260416670080588, -6.551208109652273848, -3.782341765625003571 ) ) ;
#53451=CARTESIAN_POINT ( 'NONE',  ( 185.4479166673494603, -6.668395609140176816, -3.850000000000003642 ) ) ;
#53541=CARTESIAN_POINT ( 'NONE',  ( 195.0435778713738557, 0.000000000000000000, -8.040022453829767102 ) ) ;
#53620=ORIENTED_EDGE ( 'NONE', *, *, #121353, .T. ) ;
#53720=AXIS2_PLACEMENT_3D ( 'NONE', #59377, #48239, #117591 ) ;
#53768=CARTESIAN_POINT ( 'NONE',  ( 185.6302083336747444, -4.367472073101514418, -7.564683531250002702 ) ) ;
#53770=CARTESIAN_POINT ( 'NONE',  ( 186.2135416670080588, 4.367472073101518859, -7.564683531249999149 ) ) ;
#53800=CARTESIAN_POINT ( 'NONE',  ( 186.9843750003414016, -8.734944146203032389, -1.604583208406767949E-15 ) ) ;
#53828=VERTEX_POINT ( 'NONE', #106194 ) ;
#53873=APPLICATION_CONTEXT ( 'automotive_design' ) ;
#53877=ORIENTED_EDGE ( 'NONE', *, *, #80486, .T. ) ;
#53925=DIRECTION ( 'NONE',  ( 0.000000000000000000, 1.224646799147352468E-16, 1.000000000000000000 ) ) ;
#53964=DIRECTION ( 'NONE',  ( 1.000000000000000000, -0.000000000000000000, -0.000000000000000000 ) ) ;
#54020=MECHANICAL_DESIGN_GEOMETRIC_PRESENTATION_REPRESENTATION('',(#102140),#97925);
#54027=CARTESIAN_POINT ( 'NONE',  ( 185.8177083336747444, 4.367472073101515306, 7.564683531250000925 ) ) ;
#54083=CARTESIAN_POINT ( 'NONE',  ( 186.7760416670080588, 6.551208109652274736, 3.782341765625001351 ) ) ;
#54095=VERTEX_POINT ( 'NONE', #111312 ) ;
#54215=ORIENTED_EDGE ( 'NONE', *, *, #53104, .F. ) ;
#54323=AXIS2_PLACEMENT_3D ( 'NONE', #43938, #83836, #84500 ) ;
#54336=CARTESIAN_POINT ( 'NONE',  ( 194.5000000000000000, 0.000000000000000000, 0.000000000000000000 ) ) ;
#54409=CARTESIAN_POINT ( 'NONE',  ( 186.8802083336747444, 4.367472073101515306, 7.564683531250000925 ) ) ;
#54462=CARTESIAN_POINT ( 'NONE',  ( 186.8750000000000000, 8.891194145520236347, 5.444286225454521982E-16 ) ) ;
#54534=CARTESIAN_POINT ( 'NONE',  ( 185.7395833340161175, 4.445597072760159030, 7.699999999999928235 ) ) ;
#54648=CARTESIAN_POINT ( 'NONE',  ( 186.9010416670080303, -4.367472073101519747, 7.564683531249999149 ) ) ;
#54704=CARTESIAN_POINT ( 'NONE',  ( 185.4010416670080588, -4.367472073101519747, 7.564683531249999149 ) ) ;
#54816=CIRCLE ( 'NONE', #25562, 0.5000000000000000000 ) ;
#54952=FACE_OUTER_BOUND ( 'NONE', #112440, .T. ) ;
#54972=VERTEX_POINT ( 'NONE', #44455 ) ;
#55027=FACE_OUTER_BOUND ( 'NONE', #47702, .T. ) ;
#55030=AXIS2_PLACEMENT_3D ( 'NONE', #62038, #41764, #113050 ) ;
#55062=CARTESIAN_POINT ( 'NONE',  ( 186.2135416670080872, 4.367472073101518859, -7.564683531249999149 ) ) ;
#55098=CARTESIAN_POINT ( 'NONE',  ( 186.8177083336747160, 4.367472073101515306, 7.564683531250000925 ) ) ;
#55117=CARTESIAN_POINT ( 'NONE',  ( 186.8333333333333144, 6.668395609140177704, -3.849999999999998312 ) ) ;
#55161=( BOUNDED_CURVE ( )  B_SPLINE_CURVE ( 2, ( #72104, #112666, #22366, #92363, #71428, #62286, #64194 ),
 .UNSPECIFIED., .F., .F. ) 
 B_SPLINE_CURVE_WITH_KNOTS ( ( 3, 2, 2, 3 ),
 ( 0.07142857142857149400, 0.09523809523809532995, 0.1190476190476191520, 0.1428571428571429880 ),
 .UNSPECIFIED. ) 
 CURVE ( )  GEOMETRIC_REPRESENTATION_ITEM ( )  RATIONAL_B_SPLINE_CURVE ( ( 0.9999999999999996669, 0.8660254037844390407, 1.000000000000000000, 0.8660254037844387076, 1.000000000000000000, 0.8660254037844379305, 1.000000000000000666 ) ) 
 REPRESENTATION_ITEM ( '' )  );
#55284=VERTEX_POINT ( 'NONE', #120294 ) ;
#55300=CARTESIAN_POINT ( 'NONE',  ( 184.5000000000000000, 0.000000000000000000, -7.699999999999999289 ) ) ;
#55320=CARTESIAN_POINT ( 'NONE',  ( 185.1927083336747160, 6.551208109652275624, -3.782341765624998686 ) ) ;
#55373=CARTESIAN_POINT ( 'NONE',  ( 186.2760416670080588, 6.551208109652274736, 3.782341765625001351 ) ) ;
#55488=DIRECTION ( 'NONE',  ( 1.000000000000000000, -0.000000000000000000, -0.000000000000000000 ) ) ;
#55539=DIRECTION ( 'NONE',  ( 0.000000000000000000, -0.000000000000000000, -1.000000000000000000 ) ) ;
#55560=FACE_OUTER_BOUND ( 'NONE', #5039, .T. ) ;
#55572=ORIENTED_EDGE ( 'NONE', *, *, #110172, .T. ) ;
#55624=DIRECTION ( 'NONE',  ( 1.000000000000000000, 0.000000000000000000, 0.000000000000000000 ) ) ;
#55697=CARTESIAN_POINT ( 'NONE',  ( 184.9635416670080872, -4.367472073101519747, 7.564683531249999149 ) ) ;
#55700=CARTESIAN_POINT ( 'NONE',  ( 184.5885416670080872, -6.551208109652273848, -3.782341765625003571 ) ) ;
#55948=CARTESIAN_POINT ( 'NONE',  ( 186.9635416670080303, -4.367472073101519747, 7.564683531249999149 ) ) ;
#55975=FACE_OUTER_BOUND ( 'NONE', #106140, .T. ) ;
#56000=CARTESIAN_POINT ( 'NONE',  ( 185.6510416670080303, 4.367472073101518859, -7.564683531249999149 ) ) ;
#56016=DIRECTION ( 'NONE',  ( -1.000000000000000000, 0.000000000000000000, 0.000000000000000000 ) ) ;
#56029=CARTESIAN_POINT ( 'NONE',  ( 185.5000000000000000, 0.000000000000000000, 7.700000000000000178 ) ) ;
#56137=CLOSED_SHELL ( 'NONE', ( #6996, #119013, #7002, #12005, #47034, #21334, #85328, #29069, #24387, #46124, #123627, #104998, #127169, #76353, #25927, #65525, #48372, #115425, #39012, #111285, #33928, #24746, #20525, #4934, #77923, #101654, #962, #103386, #64646, #18183, #46466, #40884, #113944, #5637, #100360, #78667 ) ) ;
#56213=CARTESIAN_POINT ( 'NONE',  ( 194.5000000000000000, 0.000000000000000000, -5.000000000000000000 ) ) ;
#56259=CARTESIAN_POINT ( 'NONE',  ( 185.2500000000000000, 9.429780353434619030E-16, -7.700000000000000178 ) ) ;
#56309=DIRECTION ( 'NONE',  ( 0.000000000000000000, 0.000000000000000000, -1.000000000000000000 ) ) ;
#56338=CARTESIAN_POINT ( 'NONE',  ( 184.0052083336747160, -6.551208109652278289, 3.782341765624995134 ) ) ;
#56341=CARTESIAN_POINT ( 'NONE',  ( 185.5052083336747444, -6.551208109652278289, 3.782341765624995134 ) ) ;
#56373=CARTESIAN_POINT ( 'NONE',  ( 186.6927083336747160, 6.551208109652275624, -3.782341765624998686 ) ) ;
#56400=ORIENTED_EDGE ( 'NONE', *, *, #6078, .T. ) ;
#56484=EDGE_LOOP ( 'NONE', ( #43300, #22670 ) ) ;
#56579=CARTESIAN_POINT ( 'NONE',  ( 185.7968750003414300, 8.734944146203032389, 5.348610694689227483E-16 ) ) ;
#56607=DIRECTION ( 'NONE',  ( 0.000000000000000000, 0.000000000000000000, -1.000000000000000000 ) ) ;
#56640=DIRECTION ( 'NONE',  ( 1.000000000000000000, 0.000000000000000000, 0.000000000000000000 ) ) ;
#56792=CARTESIAN_POINT ( 'NONE',  ( 195.0000000000000000, 0.000000000000000000, -4.000000000000000000 ) ) ;
#56793=EDGE_CURVE ( 'NONE', #8279, #120770, #72740, .T. ) ;
#56974=CARTESIAN_POINT ( 'NONE',  ( 187.4583333333333428, 4.445597072760117285, 7.699999999999999289 ) ) ;
#56977=CARTESIAN_POINT ( 'NONE',  ( 185.8802083336747444, 4.367472073101515306, 7.564683531250000925 ) ) ;
#57200=LINE ( 'NONE', #116114, #124462 ) ;
#57201=CARTESIAN_POINT ( 'NONE',  ( 187.2812500006828031, 0.000000000000000000, 7.700000000000000178 ) ) ;
#57245=CARTESIAN_POINT ( 'NONE',  ( 185.2552083336747444, 6.551208109652275624, -3.782341765624998686 ) ) ;
#57382=AXIS2_PLACEMENT_3D ( 'NONE', #94833, #35912, #124939 ) ;
#57605=CARTESIAN_POINT ( 'NONE',  ( 186.0312500006828031, 9.429780353434619030E-16, -7.700000000000000178 ) ) ;
#57620=CYLINDRICAL_SURFACE ( 'NONE', #8828, 5.000000000000000000 ) ;
#57647=CARTESIAN_POINT ( 'NONE',  ( 184.3385416670080872, 6.551208109652274736, 3.782341765625001351 ) ) ;
#57680=CARTESIAN_POINT ( 'NONE',  ( 184.5138397154228187, -7.190708303082583797, -2.674694939153578588 ) ) ;
#57700=( LENGTH_UNIT ( ) NAMED_UNIT ( * ) SI_UNIT ( .MILLI., .METRE. ) );
#57741=CARTESIAN_POINT ( 'NONE',  ( 186.0833333333333144, -6.668395609140180369, 3.849999999999994760 ) ) ;
#57906=CARTESIAN_POINT ( 'NONE',  ( 186.4635416670080872, -4.367472073101519747, 7.564683531249999149 ) ) ;
#58016=TOROIDAL_SURFACE ( 'NONE', #37086, 7.541925104783893552, 0.5000000000000000000 ) ;
#58060=COLOUR_RGB ( '', 0.66274510, 0.83137255, 0.94901961) ;
#58100=CARTESIAN_POINT ( 'NONE',  ( 184.5000000000000000, 0.000000000000000000, 0.000000000000000000 ) ) ;
#58108=ORIENTED_EDGE ( 'NONE', *, *, #39988, .T. ) ;
#58116=CARTESIAN_POINT ( 'NONE',  ( 186.6979166673494603, 6.668395609140176816, 3.850000000000000977 ) ) ;
#58129=ORIENTED_EDGE ( 'NONE', *, *, #39529, .F. ) ;
#58179=CARTESIAN_POINT ( 'NONE',  ( 194.5000000000000000, 0.000000000000000000, 0.000000000000000000 ) ) ;
#58204=CARTESIAN_POINT ( 'NONE',  ( 184.6562500006828031, 8.891194145520236347, 5.444286225454521982E-16 ) ) ;
#58214=ORIENTED_EDGE ( 'NONE', *, *, #59037, .T. ) ;
#58222=CARTESIAN_POINT ( 'NONE',  ( 185.0416666666667140, -4.445597072760063107, 7.700000000000102318 ) ) ;
#58259=VERTEX_POINT ( 'NONE', #73010 ) ;
#58299=CARTESIAN_POINT ( 'NONE',  ( 186.3750000000000284, 8.891194145520236347, 5.444286225454521982E-16 ) ) ;
#58334=CARTESIAN_POINT ( 'NONE',  ( 185.4010416670080872, -4.367472073101520635, 7.564683531249999149 ) ) ;
#58346=EDGE_LOOP ( 'NONE', ( #94924, #19026, #1082, #16597, #80886 ) ) ;
#58550=CARTESIAN_POINT ( 'NONE',  ( 184.1510416670080588, 4.367472073101518859, -7.564683531249999149 ) ) ;
#58615=DIRECTION ( 'NONE',  ( 0.000000000000000000, 0.000000000000000000, -1.000000000000000000 ) ) ;
#58753=CARTESIAN_POINT ( 'NONE',  ( 186.6562500006828316, 8.891194145520236347, 5.444286225454521982E-16 ) ) ;
#58810=CARTESIAN_POINT ( 'NONE',  ( 184.5000000000000000, 0.000000000000000000, 0.000000000000000000 ) ) ;
#58866=CARTESIAN_POINT ( 'NONE',  ( 184.5000000000000000, 0.000000000000000000, -7.699999999999999289 ) ) ;
#58923=AXIS2_PLACEMENT_3D ( 'NONE', #58100, #61320, #42320 ) ;
#58934=CARTESIAN_POINT ( 'NONE',  ( 187.2083333333333428, -4.445597072760115509, -7.700000000000001954 ) ) ;
#58957=CARTESIAN_POINT ( 'NONE',  ( 184.5000000000000000, -2.986254062820097310, -7.097343634930640022 ) ) ;
#58965=CARTESIAN_POINT ( 'NONE',  ( 184.6510416670080588, 4.367472073101518859, -7.564683531249999149 ) ) ;
#59037=EDGE_CURVE ( 'NONE', #28707, #64176, #105750, .T. ) ;
#59093=CARTESIAN_POINT ( 'NONE',  ( 185.5000000000000000, 0.000000000000000000, 7.700000000000000178 ) ) ;
#59270=DIRECTION ( 'NONE',  ( 1.000000000000000000, 0.000000000000000000, 0.000000000000000000 ) ) ;
#59377=CARTESIAN_POINT ( 'NONE',  ( 184.5000000000000000, 0.000000000000000000, 0.000000000000000000 ) ) ;
#59537=EDGE_CURVE ( 'NONE', #35519, #1307, #5816, .T. ) ;
#59605=CARTESIAN_POINT ( 'NONE',  ( 184.2083333333333144, -4.445597072760115509, -7.700000000000001954 ) ) ;
#59935=CARTESIAN_POINT ( 'NONE',  ( 184.5000000000000000, -0.3110874738271938167, 7.694949878671636156 ) ) ;
#60062=CARTESIAN_POINT ( 'NONE',  ( 186.4479166673494603, -6.668395609140176816, -3.850000000000003642 ) ) ;
#60147=ORIENTED_EDGE ( 'NONE', *, *, #27415, .F. ) ;
#60151=( BOUNDED_CURVE ( )  B_SPLINE_CURVE ( 2, ( #34836, #66193, #83897, #35466, #114022, #74738, #75364, #5974, #36760, #53800, #104815, #95028, #106128, #55098, #115267, #64262, #56373, #5338, #45287, #45933, #6595, #85827, #46548, #25617, #65554, #36106, #63636, #86478, #126417, #113364, #123817, #13869, #93734, #4049, #14505, #74095, #94362, #4674, #69411, #38029, #97590, #18383, #89071, #19017, #28868, #39349, #98877, #58334, #26924, #117864, #89706, #7264, #67460, #66829, #98232, #68772, #68123, #127068, #7913, #108701, #79259, #129021, #37400, #47215, #17060, #58965, #78621, #49164, #8546, #57680, #109344 ),
 .UNSPECIFIED., .F., .F. ) 
 B_SPLINE_CURVE_WITH_KNOTS ( ( 3, 2, 2, 2, 2, 2, 2, 2, 2, 2, 2, 2, 2, 2, 2, 2, 2, 2, 2, 2, 2, 2, 2, 2, 2, 2, 2, 2, 2, 2, 2, 2, 2, 2, 2, 3 ),
 ( 0.000000000000000000, 0.02380952380952380820, 0.04761904761904761640, 0.07142857142857142461, 0.09523809523809523281, 0.1190476190476190271, 0.1428571428571428492, 0.1666666666666666574, 0.1904761904761904656, 0.2142857142857142738, 0.2380952380952380543, 0.2619047619047619180, 0.2857142857142856984, 0.3095238095238095344, 0.3333333333333333148, 0.3571428571428571508, 0.3809523809523809312, 0.4047619047619048227, 0.4285714285714285476, 0.4523809523809523836, 0.4761904761904761085, 0.5000000000000000000, 0.5238095238095238360, 0.5476190476190476719, 0.5714285714285713969, 0.5952380952380952328, 0.6190476190476190688, 0.6428571428571429047, 0.6666666666666666297, 0.6904761904761904656, 0.7142857142857143016, 0.7380952380952382486, 0.7619047619047618625, 0.7857142857142856984, 0.8095238095238096454, 0.8172260697265570917 ),
 .UNSPECIFIED. ) 
 CURVE ( )  GEOMETRIC_REPRESENTATION_ITEM ( )  RATIONAL_B_SPLINE_CURVE ( ( 1.000000000000000000, 0.8660254037844387076, 1.000000000000000000, 0.8660254037844387076, 1.000000000000000000, 0.8660254037844387076, 1.000000000000000000, 0.8660254037844387076, 1.000000000000000000, 0.8660254037844387076, 1.000000000000000000, 0.8660254037844387076, 1.000000000000000000, 0.8660254037844387076, 1.000000000000000000, 0.8660254037844387076, 1.000000000000000000, 0.8660254037844387076, 1.000000000000000000, 0.8660254037844387076, 1.000000000000000000, 0.8660254037844387076, 1.000000000000000000, 0.8660254037844387076, 1.000000000000000000, 0.8660254037844387076, 1.000000000000000000, 0.8660254037844387076, 1.000000000000000000, 0.8660254037844387076, 1.000000000000000000, 0.8660254037844387076, 1.000000000000000000, 0.8660254037844387076, 1.000000000000000000, 0.8660254037844387076, 1.000000000000000000, 0.8660254037844387076, 1.000000000000000000, 0.8660254037844387076, 1.000000000000000000, 0.8660254037844387076, 1.000000000000000000, 0.8660254037844387076, 1.000000000000000000, 0.8660254037844387076, 1.000000000000000000, 0.8660254037844387076, 1.000000000000000000, 0.8660254037844387076, 1.000000000000000000, 0.8660254037844387076, 1.000000000000000000, 0.8660254037844387076, 1.000000000000000000, 0.8660254037844387076, 1.000000000000000000, 0.8660254037844387076, 1.000000000000000000, 0.8660254037844387076, 1.000000000000000000, 0.8660254037844387076, 1.000000000000000000, 0.8660254037844387076, 1.000000000000000000, 0.8660254037844387076, 1.000000000000000000, 0.8660254037844387076, 1.000000000000000000, 0.9566598975743678679, 0.9413604018207953894 ) ) 
 REPRESENTATION_ITEM ( '' )  );
#60250=DIRECTION ( 'NONE',  ( 1.000000000000000000, -0.000000000000000000, -0.000000000000000000 ) ) ;
#60289=ORIENTED_EDGE ( 'NONE', *, *, #87978, .F. ) ;
#60310=CARTESIAN_POINT ( 'NONE',  ( 186.7812500006828031, 0.000000000000000000, 7.700000000000000178 ) ) ;
#60424=AXIS2_PLACEMENT_3D ( 'NONE', #123588, #42481, #114415 ) ;
#60447=CARTESIAN_POINT ( 'NONE',  ( 186.0000000000000000, 0.000000000000000000, 7.700000000000000178 ) ) ;
#60490=CARTESIAN_POINT ( 'NONE',  ( 184.9635416670080872, -4.367472073101519747, 7.564683531249999149 ) ) ;
#60679=CARTESIAN_POINT ( 'NONE',  ( 184.5833333333333144, -6.668395609140180369, 3.849999999999994760 ) ) ;
#60696=CARTESIAN_POINT ( 'NONE',  ( 186.9895833340161460, -4.445597072760115509, -7.700000000000001954 ) ) ;
#60861=CARTESIAN_POINT ( 'NONE',  ( 184.9166666666666856, 6.668395609140176816, 3.850000000000000977 ) ) ;
#60885=DIRECTION ( 'NONE',  ( 0.000000000000000000, 0.000000000000000000, -1.000000000000000000 ) ) ;
#61129=CYLINDRICAL_SURFACE ( 'NONE', #19629, 7.699999999999999289 ) ;
#61320=DIRECTION ( 'NONE',  ( 1.000000000000000000, -0.000000000000000000, -0.000000000000000000 ) ) ;
#61332=CARTESIAN_POINT ( 'NONE',  ( 184.6145833340161175, 6.668395609140177704, -3.849999999999998312 ) ) ;
#61593=CARTESIAN_POINT ( 'NONE',  ( 186.6250000000000000, -8.891194145520236347, -1.633285867636356299E-15 ) ) ;
#61866=EDGE_LOOP ( 'NONE', ( #113763, #75083, #44286, #92155 ) ) ;
#61980=CARTESIAN_POINT ( 'NONE',  ( 186.9843750003414300, -8.734944146203032389, -1.604583208406768146E-15 ) ) ;
#61987=EDGE_CURVE ( 'NONE', #17533, #35519, #123346, .T. ) ;
#62038=CARTESIAN_POINT ( 'NONE',  ( 187.5000000000000000, 0.000000000000000000, 0.000000000000000000 ) ) ;
#62120=CARTESIAN_POINT ( 'NONE',  ( 195.5000000000000000, 0.000000000000000000, -5.000000000000000000 ) ) ;
#62286=CARTESIAN_POINT ( 'NONE',  ( 187.0416666666666572, -4.445597072760107515, 7.700000000000023270 ) ) ;
#62317=CARTESIAN_POINT ( 'NONE',  ( 187.3802083336747444, 4.367472073101515306, 7.564683531250000925 ) ) ;
#62356=ORIENTED_EDGE ( 'NONE', *, *, #103788, .T. ) ;
#62436=DIRECTION ( 'NONE',  ( 0.000000000000000000, 0.000000000000000000, -1.000000000000000000 ) ) ;
#62571=EDGE_CURVE ( 'NONE', #64176, #54972, #60151, .T. ) ;
#62572=CARTESIAN_POINT ( 'NONE',  ( 186.5260416670080588, -6.551208109652273848, -3.782341765625003571 ) ) ;
#62628=CARTESIAN_POINT ( 'NONE',  ( 185.8645833340161175, -6.668395609140180369, 3.849999999999994760 ) ) ;
#62691=AXIS2_PLACEMENT_3D ( 'NONE', #28293, #8621, #78028 ) ;
#62822=CARTESIAN_POINT ( 'NONE',  ( 184.5000000000000000, 0.000000000000000000, 0.000000000000000000 ) ) ;
#62827=DIRECTION ( 'NONE',  ( 1.000000000000000000, 0.000000000000000000, 0.000000000000000000 ) ) ;
#62943=CARTESIAN_POINT ( 'NONE',  ( 184.7968750003414016, 8.734944146203032389, 5.348610694689227483E-16 ) ) ;
#62946=CARTESIAN_POINT ( 'NONE',  ( 186.6718750003414016, 9.264065473108010111E-16, -7.564683531250000925 ) ) ;
#62997=AXIS2_PLACEMENT_3D ( 'NONE', #73758, #124159, #113703 ) ;
#63001=CARTESIAN_POINT ( 'NONE',  ( 185.2812500006828031, 0.000000000000000000, 7.700000000000000178 ) ) ;
#63026=VECTOR ( 'NONE', #55488, 1000.000000000000000 ) ;
#63058=AXIS2_PLACEMENT_3D ( 'NONE', #81315, #122527, #40768 ) ;
#63190=EDGE_LOOP ( 'NONE', ( #71775, #45060 ) ) ;
#63200=CARTESIAN_POINT ( 'NONE',  ( 185.5677083336747160, -4.367472073101514418, -7.564683531250002702 ) ) ;
#63204=DIRECTION ( 'NONE',  ( 1.000000000000000000, -0.000000000000000000, -0.000000000000000000 ) ) ;
#63251=CARTESIAN_POINT ( 'NONE',  ( 195.5000000000000000, 0.000000000000000000, -7.541925104783893552 ) ) ;
#63254=CARTESIAN_POINT ( 'NONE',  ( 185.1145833340161175, 6.668395609140177704, -3.849999999999998312 ) ) ;
#63311=FACE_OUTER_BOUND ( 'NONE', #119371, .T. ) ;
#63543=AXIS2_PLACEMENT_3D ( 'NONE', #95909, #6220, #56607 ) ;
#63601=CARTESIAN_POINT ( 'NONE',  ( 185.0052083336747444, -6.551208109652278289, 3.782341765624995134 ) ) ;
#63603=CARTESIAN_POINT ( 'NONE',  ( 186.6302083336747728, -4.367472073101514418, -7.564683531250002702 ) ) ;
#63636=CARTESIAN_POINT ( 'NONE',  ( 186.2760416670080588, 6.551208109652274736, 3.782341765625001351 ) ) ;
#63691=CARTESIAN_POINT ( 'NONE',  ( 184.1927083336747160, 6.551208109652275624, -3.782341765624998686 ) ) ;
#63848=CARTESIAN_POINT ( 'NONE',  ( 184.7760416670080588, 6.551208109652274736, 3.782341765625001351 ) ) ;
#63904=CARTESIAN_POINT ( 'NONE',  ( 185.1979166673494603, 6.668395609140176816, 3.850000000000000977 ) ) ;
#64176=VERTEX_POINT ( 'NONE', #66229 ) ;
#64194=CARTESIAN_POINT ( 'NONE',  ( 187.0000000000000000, 0.000000000000000000, 7.700000000000000178 ) ) ;
#64227=EDGE_CURVE ( 'NONE', #58259, #3309, #95294, .T. ) ;
#64233=CARTESIAN_POINT ( 'NONE',  ( 185.5468750003414300, -8.734944146203032389, -1.604583208406768146E-15 ) ) ;
#64262=CARTESIAN_POINT ( 'NONE',  ( 186.7343750003414016, 8.734944146203032389, 5.348610694689227483E-16 ) ) ;
#64374=EDGE_CURVE ( 'NONE', #86499, #85590, #24195, .T. ) ;
#64481=CARTESIAN_POINT ( 'NONE',  ( 185.0260416670080588, -6.551208109652273848, -3.782341765625003571 ) ) ;
#64526=AXIS2_PLACEMENT_3D ( 'NONE', #27417, #88264, #38572 ) ;
#64538=CARTESIAN_POINT ( 'NONE',  ( 186.0260416670080588, -6.551208109652273848, -3.782341765625003571 ) ) ;
#64646=ADVANCED_FACE ( 'NONE', ( #36647 ), #33781, .T. ) ;
#64751=EDGE_CURVE ( 'NONE', #32478, #41594, #42114, .T. ) ;
#64791=DIRECTION ( 'NONE',  ( 0.000000000000000000, 0.000000000000000000, -1.000000000000000000 ) ) ;
#64866=CARTESIAN_POINT ( 'NONE',  ( 187.0052083336747444, -6.551208109652278289, 3.782341765624995134 ) ) ;
#64928=ORIENTED_EDGE ( 'NONE', *, *, #126863, .T. ) ;
#65018=CARTESIAN_POINT ( 'NONE',  ( 185.0312500006828031, 9.429780353434619030E-16, -7.700000000000000178 ) ) ;
#65111=CARTESIAN_POINT ( 'NONE',  ( 185.6927083336747160, 6.551208109652275624, -3.782341765624998686 ) ) ;
#65162=CARTESIAN_POINT ( 'NONE',  ( 186.0677083336747444, -4.367472073101514418, -7.564683531250002702 ) ) ;
#65296=VERTEX_POINT ( 'NONE', #31184 ) ;
#65413=CARTESIAN_POINT ( 'NONE',  ( 184.5000000000000000, 9.429780353434619030E-16, 7.699999999999999289 ) ) ;
#65483=EDGE_CURVE ( 'NONE', #17533, #117178, #99509, .T. ) ;
#65517=CARTESIAN_POINT ( 'NONE',  ( 185.9635416670080872, -4.367472073101519747, 7.564683531249999149 ) ) ;
#65520=CARTESIAN_POINT ( 'NONE',  ( 185.2552083336747444, 6.551208109652275624, -3.782341765624998686 ) ) ;
#65525=ADVANCED_FACE ( 'NONE', ( #105547 ), #15856, .T. ) ;
#65554=CARTESIAN_POINT ( 'NONE',  ( 186.3593750003414016, 0.000000000000000000, 7.564683531250000925 ) ) ;
#65650=B_SPLINE_CURVE_WITH_KNOTS ( 'NONE', 3,
 ( #4364, #84232, #34524, #113712, #124824, #52856, #2444, #44981, #52217, #24048 ),
 .UNSPECIFIED., .F., .F.,
 ( 4, 2, 2, 2, 4 ),
 ( 1.339801017408199283E-15, 0.001880205780637580646, 0.003760411561273821219, 0.005640617341910062442, 0.007520823122546303231 ),
 .UNSPECIFIED. ) ;
#65764=CARTESIAN_POINT ( 'NONE',  ( 187.2968750003414300, 8.734944146203032389, 5.348610694689227483E-16 ) ) ;
#65821=CARTESIAN_POINT ( 'NONE',  ( 186.1093750003413732, 9.264065473108010111E-16, -7.564683531250000925 ) ) ;
#66111=EDGE_CURVE ( 'NONE', #39170, #27061, #71586, .T. ) ;
#66133=CARTESIAN_POINT ( 'NONE',  ( 194.5000000000000000, 0.000000000000000000, 0.000000000000000000 ) ) ;
#66159=CARTESIAN_POINT ( 'NONE',  ( 186.1250000000000000, -8.891194145520236347, -1.633285867636356693E-15 ) ) ;
#66162=CARTESIAN_POINT ( 'NONE',  ( 185.1302083336747728, -4.367472073101514418, -7.564683531250002702 ) ) ;
#66193=CARTESIAN_POINT ( 'NONE',  ( 187.3177083336747160, 4.367472073101515306, 7.564683531250000925 ) ) ;
#66229=CARTESIAN_POINT ( 'NONE',  ( 187.3593750003414016, 0.000000000000000000, 7.564683531250000925 ) ) ;
#66230=DIRECTION ( 'NONE',  ( 1.000000000000000000, 0.000000000000000000, 0.000000000000000000 ) ) ;
#66411=CARTESIAN_POINT ( 'NONE',  ( 186.0052083336747444, -6.551208109652278289, 3.782341765624995134 ) ) ;
#66469=CARTESIAN_POINT ( 'NONE',  ( 186.5260416670080588, -6.551208109652273848, -3.782341765625003571 ) ) ;
#66705=CARTESIAN_POINT ( 'NONE',  ( 184.6979166673494603, 6.668395609140176816, 3.850000000000000977 ) ) ;
#66708=ORIENTED_EDGE ( 'NONE', *, *, #25303, .T. ) ;
#66796=CARTESIAN_POINT ( 'NONE',  ( 186.8750000000000284, 8.891194145520236347, 5.444286225454521982E-16 ) ) ;
#66829=CARTESIAN_POINT ( 'NONE',  ( 185.1510416670080872, 4.367472073101518859, -7.564683531249999149 ) ) ;
#66852=( NAMED_UNIT ( * ) PLANE_ANGLE_UNIT ( ) SI_UNIT ( $, .RADIAN. ) );
#66890=CARTESIAN_POINT ( 'NONE',  ( 186.2500000000000000, 9.429780353434619030E-16, -7.700000000000000178 ) ) ;
#66962=CIRCLE ( 'NONE', #115078, 8.699999999999999289 ) ;
#67038=CARTESIAN_POINT ( 'NONE',  ( 186.2135416670080872, 4.367472073101518859, -7.564683531249999149 ) ) ;
#67056=( NAMED_UNIT ( * ) PLANE_ANGLE_UNIT ( ) SI_UNIT ( $, .RADIAN. ) );
#67295=EDGE_LOOP ( 'NONE', ( #11997, #18625 ) ) ;
#67341=AXIS2_PLACEMENT_3D ( 'NONE', #76763, #25717, #125845 ) ;
#67422=CARTESIAN_POINT ( 'NONE',  ( 185.9583333333333428, 4.445597072760117285, 7.699999999999999289 ) ) ;
#67460=CARTESIAN_POINT ( 'NONE',  ( 185.1927083336747160, 6.551208109652275624, -3.782341765624998686 ) ) ;
#67478=( LENGTH_UNIT ( ) NAMED_UNIT ( * ) SI_UNIT ( .MILLI., .METRE. ) );
#67536=CONICAL_SURFACE ( 'NONE', #55030, 8.699999999999999289, 0.08726646259971666819 ) ;
#67561=EDGE_CURVE ( 'NONE', #67674, #87604, #51135, .T. ) ;
#67593=VERTEX_POINT ( 'NONE', #50971 ) ;
#67674=VERTEX_POINT ( 'NONE', #53541 ) ;
#67697=CARTESIAN_POINT ( 'NONE',  ( 186.5052083336747444, -6.551208109652278289, 3.782341765624995134 ) ) ;
#67789=CARTESIAN_POINT ( 'NONE',  ( 184.4999999999999716, -3.021901993692428512, 7.049708900599269690 ) ) ;
#67826=CARTESIAN_POINT ( 'NONE',  ( 184.9895833340161175, -4.445597072760163471, -7.699999999999919353 ) ) ;
#67917=CARTESIAN_POINT ( 'NONE',  ( 187.2812500006828031, 0.000000000000000000, 7.700000000000000178 ) ) ;
#67947=ORIENTED_EDGE ( 'NONE', *, *, #125058, .F. ) ;
#68093=CARTESIAN_POINT ( 'NONE',  ( 184.4635416670080588, -4.367472073101519747, 7.564683531249999149 ) ) ;
#68123=CARTESIAN_POINT ( 'NONE',  ( 185.0260416670080588, -6.551208109652273848, -3.782341765625003571 ) ) ;
#68206=EDGE_CURVE ( 'NONE', #17430, #109569, #95223, .T. ) ;
#68222=VECTOR ( 'NONE', #15347, 1000.000000000000000 ) ;
#68349=CARTESIAN_POINT ( 'NONE',  ( 186.5885416670080872, -6.551208109652273848, -3.782341765625003571 ) ) ;
#68362=FACE_OUTER_BOUND ( 'NONE', #67295, .T. ) ;
#68558=CARTESIAN_POINT ( 'NONE',  ( 186.7395833340161175, 4.445597072760117285, 7.699999999999999289 ) ) ;
#68606=CARTESIAN_POINT ( 'NONE',  ( 186.5312500006828031, 9.429780353434619030E-16, -7.700000000000000178 ) ) ;
#68613=DIRECTION ( 'NONE',  ( 1.000000000000000000, -0.000000000000000000, -0.000000000000000000 ) ) ;
#68637=EDGE_CURVE ( 'NONE', #87604, #67674, #51497, .T. ) ;
#68706=ORIENTED_EDGE ( 'NONE', *, *, #12521, .T. ) ;
#68745=CARTESIAN_POINT ( 'NONE',  ( 184.4218750003414016, 0.000000000000000000, 7.564683531250000925 ) ) ;
#68772=CARTESIAN_POINT ( 'NONE',  ( 185.0677083336747160, -4.367472073101514418, -7.564683531250002702 ) ) ;
#68948=CARTESIAN_POINT ( 'NONE',  ( 185.8750000000000000, 8.891194145520236347, 5.444286225454521982E-16 ) ) ;
#69048=DIRECTION ( 'NONE',  ( 1.000000000000000000, 0.000000000000000000, 0.000000000000000000 ) ) ;
#69224=ORIENTED_EDGE ( 'NONE', *, *, #56793, .F. ) ;
#69252=DIRECTION ( 'NONE',  ( 0.000000000000000000, 0.000000000000000000, -1.000000000000000000 ) ) ;
#69267=DIRECTION ( 'NONE',  ( 0.000000000000000000, 0.000000000000000000, -1.000000000000000000 ) ) ;
#69281=( BOUNDED_CURVE ( )  B_SPLINE_CURVE ( 2, ( #81308, #2080, #32869, #2728, #72773, #121223, #51852, #11909, #71469, #122519, #123165, #83867, #42694, #91123, #31562, #53136, #91762, #23030, #62946, #63603, #82602, #102855, #93068, #3380, #23670, #43327, #33507, #103524, #13836, #53770, #46517, #74058, #5942, #96912, #26256, #95635, #35436, #56977, #114617, #75336, #6567, #74703, #25584, #125090, #86445, #125713, #56341, #45895, #7229, #47187, #14469, #94327, #65520, #36729, #85164, #66162, #106098, #34143, #34800, #4640, #115233, #85800, #105458, #16396, #15768, #113988, #104784, #123781, #55700, #76641, #24314, #96256, #36070 ),
 .UNSPECIFIED., .F., .F. ) 
 B_SPLINE_CURVE_WITH_KNOTS ( ( 3, 2, 2, 2, 2, 2, 2, 2, 2, 2, 2, 2, 2, 2, 2, 2, 2, 2, 2, 2, 2, 2, 2, 2, 2, 2, 2, 2, 2, 2, 2, 2, 2, 2, 2, 2, 3 ),
 ( 0.000000000000000000, 0.02380952380952380820, 0.04761904761904761640, 0.07142857142857142461, 0.09523809523809523281, 0.1190476190476190410, 0.1428571428571428492, 0.1666666666666666574, 0.1904761904761904656, 0.2142857142857142461, 0.2380952380952380820, 0.2619047619047619180, 0.2857142857142856984, 0.3095238095238095344, 0.3333333333333333148, 0.3571428571428571508, 0.3809523809523809312, 0.4047619047619048227, 0.4285714285714284921, 0.4523809523809523836, 0.4761904761904761640, 0.5000000000000000000, 0.5238095238095238360, 0.5476190476190476719, 0.5714285714285713969, 0.5952380952380952328, 0.6190476190476190688, 0.6428571428571430157, 0.6666666666666666297, 0.6904761904761903546, 0.7142857142857143016, 0.7380952380952381375, 0.7619047619047618625, 0.7857142857142856984, 0.8095238095238096454, 0.8333333333333333703, 0.8350034827724532871 ),
 .UNSPECIFIED. ) 
 CURVE ( )  GEOMETRIC_REPRESENTATION_ITEM ( )  RATIONAL_B_SPLINE_CURVE ( ( 1.000000000000000000, 0.8660254037844387076, 1.000000000000000000, 0.8660254037844387076, 1.000000000000000000, 0.8660254037844387076, 1.000000000000000000, 0.8660254037844387076, 1.000000000000000000, 0.8660254037844387076, 1.000000000000000000, 0.8660254037844387076, 1.000000000000000000, 0.8660254037844387076, 1.000000000000000000, 0.8660254037844387076, 1.000000000000000000, 0.8660254037844387076, 1.000000000000000000, 0.8660254037844387076, 1.000000000000000000, 0.8660254037844387076, 1.000000000000000000, 0.8660254037844387076, 1.000000000000000000, 0.8660254037844387076, 1.000000000000000000, 0.8660254037844387076, 1.000000000000000000, 0.8660254037844387076, 1.000000000000000000, 0.8660254037844387076, 1.000000000000000000, 0.8660254037844387076, 1.000000000000000000, 0.8660254037844387076, 1.000000000000000000, 0.8660254037844387076, 1.000000000000000000, 0.8660254037844387076, 1.000000000000000000, 0.8660254037844387076, 1.000000000000000000, 0.8660254037844387076, 1.000000000000000000, 0.8660254037844387076, 1.000000000000000000, 0.8660254037844387076, 1.000000000000000000, 0.8660254037844387076, 1.000000000000000000, 0.8660254037844387076, 1.000000000000000000, 0.8660254037844387076, 1.000000000000000000, 0.8660254037844387076, 1.000000000000000000, 0.8660254037844387076, 1.000000000000000000, 0.8660254037844387076, 1.000000000000000000, 0.8660254037844387076, 1.000000000000000000, 0.8660254037844387076, 1.000000000000000000, 0.8660254037844387076, 1.000000000000000000, 0.8660254037844387076, 1.000000000000000000, 0.8660254037844387076, 1.000000000000000000, 0.9906021809375190612, 0.9825228059028749961 ) ) 
 REPRESENTATION_ITEM ( '' )  );
#69288=PRODUCT_DEFINITION_FORMATION_WITH_SPECIFIED_SOURCE ( 'ANY', '', #7300, .NOT_KNOWN. ) ;
#69291=EDGE_CURVE ( 'NONE', #109689, #70723, #11956, .T. ) ;
#69359=CARTESIAN_POINT ( 'NONE',  ( 186.3645833340161175, -6.668395609140180369, 3.849999999999994760 ) ) ;
#69382=CARTESIAN_POINT ( 'NONE',  ( 184.4583333333333428, 4.445597072760117285, 7.699999999999999289 ) ) ;
#69411=CARTESIAN_POINT ( 'NONE',  ( 185.7760416670080588, 6.551208109652274736, 3.782341765625001351 ) ) ;
#69447=CARTESIAN_POINT ( 'NONE',  ( 186.7500000000000000, 9.429780353434619030E-16, -7.700000000000000178 ) ) ;
#69663=SURFACE_STYLE_USAGE ( .BOTH. , #78209 ) ;
#69778=CARTESIAN_POINT ( 'NONE',  ( 186.4166666666666856, 6.668395609140176816, 3.850000000000000977 ) ) ;
#69797=CARTESIAN_POINT ( 'NONE',  ( 186.9843750003414300, -8.734944146203032389, -1.604583208406768146E-15 ) ) ;
#69842=CARTESIAN_POINT ( 'NONE',  ( 184.6250000000000000, -8.891194145520236347, -1.633285867636356299E-15 ) ) ;
#69862=CARTESIAN_POINT ( 'NONE',  ( 187.1979166673494603, 6.668395609140176816, 3.850000000000000977 ) ) ;
#70184=VERTEX_POINT ( 'NONE', #57605 ) ;
#70228=DIRECTION ( 'NONE',  ( 1.000000000000000000, -0.000000000000000000, -0.000000000000000000 ) ) ;
#70294=CARTESIAN_POINT ( 'NONE',  ( 184.0468750003414300, -8.734944146203032389, -1.604583208406768146E-15 ) ) ;
#70426=CARTESIAN_POINT ( 'NONE',  ( 186.3750000000000000, 8.891194145520236347, 5.444286225454521982E-16 ) ) ;
#70496=CARTESIAN_POINT ( 'NONE',  ( 186.1562500006828031, 8.891194145520236347, 5.444286225454521982E-16 ) ) ;
#70524=VERTEX_POINT ( 'NONE', #102040 ) ;
#70689=FACE_OUTER_BOUND ( 'NONE', #34350, .T. ) ;
#70723=VERTEX_POINT ( 'NONE', #20101 ) ;
#70831=CARTESIAN_POINT ( 'NONE',  ( 187.2968750003414300, 8.734944146203032389, 5.348610694689227483E-16 ) ) ;
#70886=DIRECTION ( 'NONE',  ( 1.000000000000000000, -0.000000000000000000, -0.000000000000000000 ) ) ;
#70933=CARTESIAN_POINT ( 'NONE',  ( 184.3802083336747444, 4.367472073101515306, 7.564683531250000925 ) ) ;
#71026=CARTESIAN_POINT ( 'NONE',  ( 184.5000000000000000, 0.000000000000000000, 7.700000000000000178 ) ) ;
#71122=CARTESIAN_POINT ( 'NONE',  ( 184.6666666666666856, -6.668395609140176816, -3.850000000000003642 ) ) ;
#71137=CARTESIAN_POINT ( 'NONE',  ( 187.2343750003414016, 8.734944146203032389, 5.348610694689227483E-16 ) ) ;
#71255=CARTESIAN_POINT ( 'NONE',  ( 195.0000000000000000, 4.898587196589412829E-16, 4.000000000000000000 ) ) ;
#71428=CARTESIAN_POINT ( 'NONE',  ( 187.0833333333333144, -6.668395609140180369, 3.849999999999994760 ) ) ;
#71469=CARTESIAN_POINT ( 'NONE',  ( 187.0885416670080872, -6.551208109652273848, -3.782341765625003571 ) ) ;
#71570=CARTESIAN_POINT ( 'NONE',  ( 183.9218750003414016, 0.000000000000000000, 7.564683531250000925 ) ) ;
#71586=CIRCLE ( 'NONE', #38138, 7.699999999999999289 ) ;
#71630=FACE_OUTER_BOUND ( 'NONE', #50005, .T. ) ;
#71690=ORIENTED_EDGE ( 'NONE', *, *, #64374, .F. ) ;
#71732=CARTESIAN_POINT ( 'NONE',  ( 187.1927083336747160, 6.551208109652275624, -3.782341765624998686 ) ) ;
#71742=FACE_OUTER_BOUND ( 'NONE', #40093, .T. ) ;
#71775=ORIENTED_EDGE ( 'NONE', *, *, #27677, .F. ) ;
#71797=CARTESIAN_POINT ( 'NONE',  ( 185.3645833340161175, -6.668395609140180369, 3.849999999999994760 ) ) ;
#72104=CARTESIAN_POINT ( 'NONE',  ( 187.2500000000000000, 9.429780353434619030E-16, -7.700000000000000178 ) ) ;
#72168=DIRECTION ( 'NONE',  ( 0.000000000000000000, 0.000000000000000000, -1.000000000000000000 ) ) ;
#72186=ORIENTED_EDGE ( 'NONE', *, *, #129551, .F. ) ;
#72392=CARTESIAN_POINT ( 'NONE',  ( 186.4010416670080588, -4.367472073101519747, 7.564683531249999149 ) ) ;
#72441=CARTESIAN_POINT ( 'NONE',  ( 184.5312500006828031, 9.429780353434619030E-16, -7.700000000000000178 ) ) ;
#72483=CARTESIAN_POINT ( 'NONE',  ( 184.5000000000000000, 9.429780353434619030E-16, 7.699999999999999289 ) ) ;
#72740=( BOUNDED_CURVE ( )  B_SPLINE_CURVE ( 2, ( #109023, #67826, #79590, #88084, #16770, #88763, #7612 ),
 .UNSPECIFIED., .F., .F. ) 
 B_SPLINE_CURVE_WITH_KNOTS ( ( 3, 2, 2, 3 ),
 ( 0.6428571428571433488, 0.6666666666666670737, 0.6904761904761910207, 0.7142857142857148567 ),
 .UNSPECIFIED. ) 
 CURVE ( )  GEOMETRIC_REPRESENTATION_ITEM ( )  RATIONAL_B_SPLINE_CURVE ( ( 0.9999999999999974465, 0.8660254037844412611, 1.000000000000000000, 0.8660254037844387076, 1.000000000000000000, 0.8660254037844355990, 1.000000000000003109 ) ) 
 REPRESENTATION_ITEM ( '' )  );
#72761=EDGE_CURVE ( 'NONE', #70524, #39170, #102787, .T. ) ;
#72769=CARTESIAN_POINT ( 'NONE',  ( 186.9218750003414016, 0.000000000000000000, 7.564683531250000925 ) ) ;
#72773=CARTESIAN_POINT ( 'NONE',  ( 187.2552083336747444, 6.551208109652275624, -3.782341765624998686 ) ) ;
#72808=DIRECTION ( 'NONE',  ( 0.000000000000000000, 0.000000000000000000, 1.000000000000000000 ) ) ;
#72854=CARTESIAN_POINT ( 'NONE',  ( 184.9583333333332860, 4.445597072760175905, 7.699999999999896261 ) ) ;
#72860=CARTESIAN_POINT ( 'NONE',  ( 184.3593750003413732, 0.000000000000000000, 7.564683531250000925 ) ) ;
#72930=CIRCLE ( 'NONE', #98056, 5.200000000000000178 ) ;
#73010=CARTESIAN_POINT ( 'NONE',  ( 187.0312500006828031, 9.429780353434619030E-16, -7.700000000000000178 ) ) ;
#73019=CARTESIAN_POINT ( 'NONE',  ( 185.7343750003414016, 8.734944146203032389, 5.348610694689227483E-16 ) ) ;
#73078=CARTESIAN_POINT ( 'NONE',  ( 184.0729166673494603, 4.445597072760120838, -7.699999999999998401 ) ) ;
#73294=AXIS2_PLACEMENT_3D ( 'NONE', #105383, #123093, #24888 ) ;
#73401=CARTESIAN_POINT ( 'NONE',  ( 184.5885416670080872, -6.551208109652273848, -3.782341765625003571 ) ) ;
#73452=CARTESIAN_POINT ( 'NONE',  ( 187.0000000000000000, 0.000000000000000000, 7.700000000000000178 ) ) ;
#73491=( BOUNDED_CURVE ( )  B_SPLINE_CURVE ( 2, ( #76543, #87632, #66705, #58204, #127571, #77811, #117726 ),
 .UNSPECIFIED., .F., .F. ) 
 B_SPLINE_CURVE_WITH_KNOTS ( ( 3, 2, 2, 3 ),
 ( 0.7142857142857148567, 0.7380952380952386926, 0.7619047619047624176, 0.7857142857142862535 ),
 .UNSPECIFIED. ) 
 CURVE ( )  GEOMETRIC_REPRESENTATION_ITEM ( )  RATIONAL_B_SPLINE_CURVE ( ( 0.9999999999999968914, 0.8660254037844418162, 1.000000000000000000, 0.8660254037844387076, 1.000000000000000000, 0.8660254037844355990, 1.000000000000003109 ) ) 
 REPRESENTATION_ITEM ( '' )  );
#73518=EDGE_CURVE ( 'NONE', #108189, #82135, #109439, .T. ) ;
#73550=CARTESIAN_POINT ( 'NONE',  ( 184.5000000000000000, 0.000000000000000000, 0.000000000000000000 ) ) ;
#73590=ORIENTED_EDGE ( 'NONE', *, *, #30995, .F. ) ;
#73600=TOROIDAL_SURFACE ( 'NONE', #23428, 7.541925104783893552, 0.5000000000000000000 ) ;
#73647=CARTESIAN_POINT ( 'NONE',  ( 184.9427083336747160, -6.551208109652278289, 3.782341765624995134 ) ) ;
#73659=ORIENTED_EDGE ( 'NONE', *, *, #51179, .T. ) ;
#73705=CARTESIAN_POINT ( 'NONE',  ( 187.2760416670080588, 6.551208109652274736, 3.782341765625001351 ) ) ;
#73758=CARTESIAN_POINT ( 'NONE',  ( 194.5000000000000000, 0.000000000000000000, 0.000000000000000000 ) ) ;
#74056=CARTESIAN_POINT ( 'NONE',  ( 187.1302083336747444, -4.367472073101514418, -7.564683531250002702 ) ) ;
#74058=CARTESIAN_POINT ( 'NONE',  ( 186.1302083336747444, -4.367472073101514418, -7.564683531250002702 ) ) ;
#74095=CARTESIAN_POINT ( 'NONE',  ( 185.9010416670080303, -4.367472073101520635, 7.564683531249999149 ) ) ;
#74149=CARTESIAN_POINT ( 'NONE',  ( 184.6927083336747160, 6.551208109652275624, -3.782341765624998686 ) ) ;
#74159=DIRECTION ( 'NONE',  ( -1.000000000000000000, -0.000000000000000000, -0.000000000000000000 ) ) ;
#74315=CARTESIAN_POINT ( 'NONE',  ( 185.3593750003413732, 0.000000000000000000, 7.564683531250000925 ) ) ;
#74366=CARTESIAN_POINT ( 'NONE',  ( 186.4843750003414016, -8.734944146203032389, -1.604583208406768146E-15 ) ) ;
#74511=DIRECTION ( 'NONE',  ( 1.000000000000000000, 0.000000000000000000, 0.000000000000000000 ) ) ;
#74614=DIRECTION ( 'NONE',  ( 1.000000000000000000, 0.000000000000000000, 0.000000000000000000 ) ) ;
#74677=ORIENTED_EDGE ( 'NONE', *, *, #52602, .F. ) ;
#74702=CARTESIAN_POINT ( 'NONE',  ( 185.5885416670080872, -6.551208109652273848, -3.782341765625003571 ) ) ;
#74703=CARTESIAN_POINT ( 'NONE',  ( 185.7135416670080588, 4.367472073101518859, -7.564683531249999149 ) ) ;
#74738=CARTESIAN_POINT ( 'NONE',  ( 187.1510416670080588, 4.367472073101518859, -7.564683531249999149 ) ) ;
#74956=CARTESIAN_POINT ( 'NONE',  ( 184.2760416670080588, 6.551208109652274736, 3.782341765625001351 ) ) ;
#75015=CARTESIAN_POINT ( 'NONE',  ( 185.1093750003413732, 9.264065473108010111E-16, -7.564683531250000925 ) ) ;
#75068=ORIENTED_EDGE ( 'NONE', *, *, #16235, .T. ) ;
#75083=ORIENTED_EDGE ( 'NONE', *, *, #68637, .T. ) ;
#75334=CARTESIAN_POINT ( 'NONE',  ( 185.2968750003414300, 8.734944146203032389, 5.348610694689227483E-16 ) ) ;
#75336=CARTESIAN_POINT ( 'NONE',  ( 185.7968750003414300, 8.734944146203032389, 5.348610694689227483E-16 ) ) ;
#75364=CARTESIAN_POINT ( 'NONE',  ( 187.1093750003414016, 9.264065473108010111E-16, -7.564683531250000925 ) ) ;
#75476=VECTOR ( 'NONE', #76387, 1000.000000000000000 ) ;
#75582=CARTESIAN_POINT ( 'NONE',  ( 184.1927083336747160, 6.551208109652275624, -3.782341765624998686 ) ) ;
#75602=LINE ( 'NONE', #4922, #114471 ) ;
#75634=CARTESIAN_POINT ( 'NONE',  ( 184.9427083336747160, -6.551208109652278289, 3.782341765624995134 ) ) ;
#75850=FACE_OUTER_BOUND ( 'NONE', #92414, .T. ) ;
#75896=CARTESIAN_POINT ( 'NONE',  ( 195.5000000000000000, 0.000000000000000000, 0.000000000000000000 ) ) ;
#75986=CARTESIAN_POINT ( 'NONE',  ( 184.3802083336747444, 4.367472073101515306, 7.564683531250000925 ) ) ;
#76180=( BOUNDED_SURFACE ( )  B_SPLINE_SURFACE ( 1, 2, ( 
 ( #39724, #82199, #81551, #121458, #71732, #40352, #29244, #80269, #119528, #69797, #19390, #54648, #114863, #122765, #102478, #25194, #103121, #114235, #13440, #93953, #62572, #122132, #32482, #72392, #112306, #33117, #92658, #22646, #12787, #4904, #52730, #112944, #2996, #23257, #44192, #84117, #42947, #54027, #82858, #73019, #65111, #123397, #105040, #63200, #53388, #93308, #94578, #15362, #74315, #124046, #3631, #24562, #55320, #43580, #83499, #33737, #64481, #95244, #73647, #113592, #45510, #23930, #63848, #103775, #14076, #34408, #5554, #4252, #104412, #14718, #44861, #84774, #124704, #35049, #74956, #127918, #75582, #58550, #115498, #38262, #86703, #77522, #27144, #78185, #106969 ),
 ( #25855, #35678, #97807, #65764, #76250, #105710, #116152, #7489, #47435, #16013, #17287, #55948, #36341, #118090, #126638, #28439, #95885, #6192, #46134, #17958, #68349, #37619, #67697, #57906, #86035, #108275, #125971, #117419, #125343, #67038, #18606, #26507, #8132, #87331, #66411, #127287, #106344, #16653, #27772, #56579, #98440, #8765, #36969, #107638, #96500, #76889, #48082, #6822, #116794, #87967, #85413, #46791, #57245, #97169, #81411, #31036, #49380, #10080, #40856, #60490, #89919, #30384, #80112, #78842, #91219, #48727, #51315, #80763, #120682, #41501, #29716, #99113, #128593, #70933, #21850, #50029, #1536, #31654, #89285, #79479, #121317, #70294, #119374, #40190, #71570 ) ),
 .UNSPECIFIED., .F., .F., .F. ) 
 B_SPLINE_SURFACE_WITH_KNOTS ( ( 2, 2 ),
 ( 3, 2, 2, 2, 2, 2, 2, 2, 2, 2, 2, 2, 2, 2, 2, 2, 2, 2, 2, 2, 2, 2, 2, 2, 2, 2, 2, 2, 2, 2, 2, 2, 2, 2, 2, 2, 2, 2, 2, 2, 2, 2, 3 ),
 ( 0.000000000000000000, 1.000000000000000000 ),
 ( 0.000000000000000000, 0.02380952380952380820, 0.04761904761904761640, 0.07142857142857142461, 0.09523809523809523281, 0.1190476190476190410, 0.1428571428571428492, 0.1666666666666666574, 0.1904761904761904656, 0.2142857142857142738, 0.2380952380952380820, 0.2619047619047619180, 0.2857142857142856984, 0.3095238095238095344, 0.3333333333333333148, 0.3571428571428571508, 0.3809523809523809312, 0.4047619047619047672, 0.4285714285714285476, 0.4523809523809523836, 0.4761904761904761640, 0.5000000000000000000, 0.5238095238095238360, 0.5476190476190476719, 0.5714285714285713969, 0.5952380952380952328, 0.6190476190476190688, 0.6428571428571429047, 0.6666666666666666297, 0.6904761904761904656, 0.7142857142857143016, 0.7380952380952381375, 0.7619047619047618625, 0.7857142857142856984, 0.8095238095238095344, 0.8333333333333333703, 0.8571428571428570953, 0.8809523809523809312, 0.9047619047619047672, 0.9285714285714286031, 0.9523809523809523281, 0.9761904761904761640, 1.000000000000000000 ),
 .UNSPECIFIED. ) 
 GEOMETRIC_REPRESENTATION_ITEM ( )  RATIONAL_B_SPLINE_SURFACE ( (
 ( 1.000000000000000000, 0.8660254037844387076, 1.000000000000000000, 0.8660254037844387076, 1.000000000000000000, 0.8660254037844387076, 1.000000000000000000, 0.8660254037844387076, 1.000000000000000000, 0.8660254037844387076, 1.000000000000000000, 0.8660254037844387076, 1.000000000000000000, 0.8660254037844387076, 1.000000000000000000, 0.8660254037844387076, 1.000000000000000000, 0.8660254037844387076, 1.000000000000000000, 0.8660254037844387076, 1.000000000000000000, 0.8660254037844387076, 1.000000000000000000, 0.8660254037844387076, 1.000000000000000000, 0.8660254037844387076, 1.000000000000000000, 0.8660254037844387076, 1.000000000000000000, 0.8660254037844387076, 1.000000000000000000, 0.8660254037844387076, 1.000000000000000000, 0.8660254037844387076, 1.000000000000000000, 0.8660254037844387076, 1.000000000000000000, 0.8660254037844387076, 1.000000000000000000, 0.8660254037844387076, 1.000000000000000000, 0.8660254037844387076, 1.000000000000000000, 0.8660254037844387076, 1.000000000000000000, 0.8660254037844387076, 1.000000000000000000, 0.8660254037844387076, 1.000000000000000000, 0.8660254037844387076, 1.000000000000000000, 0.8660254037844387076, 1.000000000000000000, 0.8660254037844387076, 1.000000000000000000, 0.8660254037844387076, 1.000000000000000000, 0.8660254037844387076, 1.000000000000000000, 0.8660254037844387076, 1.000000000000000000, 0.8660254037844387076, 1.000000000000000000, 0.8660254037844387076, 1.000000000000000000, 0.8660254037844387076, 1.000000000000000000, 0.8660254037844387076, 1.000000000000000000, 0.8660254037844387076, 1.000000000000000000, 0.8660254037844387076, 1.000000000000000000, 0.8660254037844387076, 1.000000000000000000, 0.8660254037844387076, 1.000000000000000000, 0.8660254037844387076, 1.000000000000000000, 0.8660254037844387076, 1.000000000000000000, 0.8660254037844387076, 1.000000000000000000, 0.8660254037844387076, 1.000000000000000000),
 ( 1.000000000000000000, 0.8660254037844387076, 1.000000000000000000, 0.8660254037844387076, 1.000000000000000000, 0.8660254037844387076, 1.000000000000000000, 0.8660254037844387076, 1.000000000000000000, 0.8660254037844387076, 1.000000000000000000, 0.8660254037844387076, 1.000000000000000000, 0.8660254037844387076, 1.000000000000000000, 0.8660254037844387076, 1.000000000000000000, 0.8660254037844387076, 1.000000000000000000, 0.8660254037844387076, 1.000000000000000000, 0.8660254037844387076, 1.000000000000000000, 0.8660254037844387076, 1.000000000000000000, 0.8660254037844387076, 1.000000000000000000, 0.8660254037844387076, 1.000000000000000000, 0.8660254037844387076, 1.000000000000000000, 0.8660254037844387076, 1.000000000000000000, 0.8660254037844387076, 1.000000000000000000, 0.8660254037844387076, 1.000000000000000000, 0.8660254037844387076, 1.000000000000000000, 0.8660254037844387076, 1.000000000000000000, 0.8660254037844387076, 1.000000000000000000, 0.8660254037844387076, 1.000000000000000000, 0.8660254037844387076, 1.000000000000000000, 0.8660254037844387076, 1.000000000000000000, 0.8660254037844387076, 1.000000000000000000, 0.8660254037844387076, 1.000000000000000000, 0.8660254037844387076, 1.000000000000000000, 0.8660254037844387076, 1.000000000000000000, 0.8660254037844387076, 1.000000000000000000, 0.8660254037844387076, 1.000000000000000000, 0.8660254037844387076, 1.000000000000000000, 0.8660254037844387076, 1.000000000000000000, 0.8660254037844387076, 1.000000000000000000, 0.8660254037844387076, 1.000000000000000000, 0.8660254037844387076, 1.000000000000000000, 0.8660254037844387076, 1.000000000000000000, 0.8660254037844387076, 1.000000000000000000, 0.8660254037844387076, 1.000000000000000000, 0.8660254037844387076, 1.000000000000000000, 0.8660254037844387076, 1.000000000000000000, 0.8660254037844387076, 1.000000000000000000, 0.8660254037844387076, 1.000000000000000000) ) ) 
 REPRESENTATION_ITEM ( '' )  SURFACE ( )  );
#76225=LINE ( 'NONE', #45484, #44198 ) ;
#76250=CARTESIAN_POINT ( 'NONE',  ( 187.2552083336747444, 6.551208109652275624, -3.782341765624998686 ) ) ;
#76258=VECTOR ( 'NONE', #96844, 1000.000000000000000 ) ;
#76303=CARTESIAN_POINT ( 'NONE',  ( 185.9010416670080303, -4.367472073101519747, 7.564683531249999149 ) ) ;
#76353=ADVANCED_FACE ( 'NONE', ( #100880 ), #129096, .T. ) ;
#76387=DIRECTION ( 'NONE',  ( 1.000000000000000000, -0.000000000000000000, -0.000000000000000000 ) ) ;
#76464=DIRECTION ( 'NONE',  ( 0.000000000000000000, 0.000000000000000000, 1.000000000000000000 ) ) ;
#76543=CARTESIAN_POINT ( 'NONE',  ( 184.7812500006828031, 0.000000000000000000, 7.700000000000000178 ) ) ;
#76638=CARTESIAN_POINT ( 'NONE',  ( 184.0885416670080872, -6.551208109652273848, -3.782341765625003571 ) ) ;
#76641=CARTESIAN_POINT ( 'NONE',  ( 184.5468750003414300, -8.734944146203032389, -1.604583208406767949E-15 ) ) ;
#76763=CARTESIAN_POINT ( 'NONE',  ( 195.5000000000000000, 0.000000000000000000, 0.000000000000000000 ) ) ;
#76850=CARTESIAN_POINT ( 'NONE',  ( 187.2395833340161460, 4.445597072760117285, 7.700000000000001066 ) ) ;
#76889=CARTESIAN_POINT ( 'NONE',  ( 185.5468750003414300, -8.734944146203032389, -1.604583208406768146E-15 ) ) ;
#77000=COLOUR_RGB ( '', 0.66274510, 0.83137255, 0.94901961) ;
#77197=CARTESIAN_POINT ( 'NONE',  ( 195.0000000000000000, 0.000000000000000000, 0.000000000000000000 ) ) ;
#77241=ORIENTED_EDGE ( 'NONE', *, *, #19986, .F. ) ;
#77278=CARTESIAN_POINT ( 'NONE',  ( 187.3750000000000000, 8.891194145520236347, 5.444286225454521982E-16 ) ) ;
#77334=AXIS2_PLACEMENT_3D ( 'NONE', #20986, #41291, #80565 ) ;
#77351=PRODUCT_DEFINITION_SHAPE ( 'NONE', 'NONE',  #98041 ) ;
#77509=ORIENTED_EDGE ( 'NONE', *, *, #64227, .F. ) ;
#77522=CARTESIAN_POINT ( 'NONE',  ( 183.9843750003414016, -8.734944146203032389, -1.604583208406768146E-15 ) ) ;
#77599=CARTESIAN_POINT ( 'NONE',  ( 184.5000000000000000, -4.107493067966395017, 6.449889041236108511 ) ) ;
#77811=CARTESIAN_POINT ( 'NONE',  ( 184.5729166673494888, 4.445597072760062218, -7.700000000000102318 ) ) ;
#77913=CARTESIAN_POINT ( 'NONE',  ( 186.7083333333333428, -4.445597072760115509, -7.700000000000001954 ) ) ;
#77923=ADVANCED_FACE ( 'NONE', ( #27481 ), #57620, .F. ) ;
#77967=SURFACE_STYLE_FILL_AREA ( #38053 ) ;
#78028=DIRECTION ( 'NONE',  ( 0.000000000000000000, 0.000000000000000000, -1.000000000000000000 ) ) ;
#78050=CARTESIAN_POINT ( 'NONE',  ( 195.0000000000000000, 9.236194438982661209E-16, 7.541925104783893552 ) ) ;
#78185=CARTESIAN_POINT ( 'NONE',  ( 183.9010416670080588, -4.367472073101519747, 7.564683531249999149 ) ) ;
#78209=SURFACE_SIDE_STYLE ('',( #117440 ) ) ;
#78308=ORIENTED_EDGE ( 'NONE', *, *, #3024, .F. ) ;
#78326=ORIENTED_EDGE ( 'NONE', *, *, #59037, .F. ) ;
#78592=CARTESIAN_POINT ( 'NONE',  ( 185.6666666666666856, -6.668395609140176816, -3.850000000000003642 ) ) ;
#78621=CARTESIAN_POINT ( 'NONE',  ( 184.6093750003413732, 9.264065473108010111E-16, -7.564683531250000925 ) ) ;
#78667=ADVANCED_FACE ( 'NONE', ( #18816 ), #86876, .T. ) ;
#78842=CARTESIAN_POINT ( 'NONE',  ( 184.7968750003414016, 8.734944146203032389, 5.348610694689227483E-16 ) ) ;
#78909=CIRCLE ( 'NONE', #49668, 5.000000000000000000 ) ;
#79050=CARTESIAN_POINT ( 'NONE',  ( 186.7812500006828031, 0.000000000000000000, 7.700000000000000178 ) ) ;
#79106=CYLINDRICAL_SURFACE ( 'NONE', #32047, 7.699999999999999289 ) ;
#79121=DIRECTION ( 'NONE',  ( -1.000000000000000000, -0.000000000000000000, -0.000000000000000000 ) ) ;
#79209=CARTESIAN_POINT ( 'NONE',  ( 186.4479166673494603, -6.668395609140176816, -3.850000000000003642 ) ) ;
#79226=CARTESIAN_POINT ( 'NONE',  ( 184.5416666666666572, -4.445597072760122614, 7.699999999999998401 ) ) ;
#79259=CARTESIAN_POINT ( 'NONE',  ( 184.8593750003413732, 0.000000000000000000, 7.564683531250000925 ) ) ;
#79277=FILL_AREA_STYLE_COLOUR ( '', #77000 ) ;
#79368=ORIENTED_EDGE ( 'NONE', *, *, #65483, .F. ) ;
#79479=CARTESIAN_POINT ( 'NONE',  ( 184.1302083336747160, -4.367472073101514418, -7.564683531250002702 ) ) ;
#79590=CARTESIAN_POINT ( 'NONE',  ( 184.9479166673494603, -6.668395609140176816, -3.850000000000003642 ) ) ;
#79758=VERTEX_POINT ( 'NONE', #47541 ) ;
#80112=CARTESIAN_POINT ( 'NONE',  ( 184.8385416670080872, 6.551208109652274736, 3.782341765625001351 ) ) ;
#80117=DIRECTION ( 'NONE',  ( 0.000000000000000000, 0.000000000000000000, -1.000000000000000000 ) ) ;
#80126=FACE_OUTER_BOUND ( 'NONE', #51809, .T. ) ;
#80254=CARTESIAN_POINT ( 'NONE',  ( 186.4583333333333428, 4.445597072760147483, 7.699999999999948663 ) ) ;
#80269=CARTESIAN_POINT ( 'NONE',  ( 187.0677083336747444, -4.367472073101514418, -7.564683531250002702 ) ) ;
#80311=DIRECTION ( 'NONE',  ( 0.000000000000000000, 0.000000000000000000, -1.000000000000000000 ) ) ;
#80331=CARTESIAN_POINT ( 'NONE',  ( 186.4062500006828031, -8.891194145520236347, -1.633285867636356693E-15 ) ) ;
#80341=EDGE_CURVE ( 'NONE', #70524, #120770, #57200, .T. ) ;
#80395=ORIENTED_EDGE ( 'NONE', *, *, #105424, .T. ) ;
#80486=EDGE_CURVE ( 'NONE', #97220, #86499, #33386, .T. ) ;
#80565=DIRECTION ( 'NONE',  ( 0.000000000000000000, 0.000000000000000000, -1.000000000000000000 ) ) ;
#80665=CARTESIAN_POINT ( 'NONE',  ( 187.4218750003414016, 0.000000000000000000, 7.564683531250000925 ) ) ;
#80718=DIRECTION ( 'NONE',  ( 1.000000000000000000, 0.000000000000000000, 0.000000000000000000 ) ) ;
#80763=CARTESIAN_POINT ( 'NONE',  ( 184.6302083336747444, -4.367472073101514418, -7.564683531250002702 ) ) ;
#80784=DIRECTION ( 'NONE',  ( 1.000000000000000000, -0.000000000000000000, -0.000000000000000000 ) ) ;
#80886=ORIENTED_EDGE ( 'NONE', *, *, #52059, .T. ) ;
#80971=CARTESIAN_POINT ( 'NONE',  ( 184.2812500006828031, 0.000000000000000000, 7.700000000000000178 ) ) ;
#81156=CARTESIAN_POINT ( 'NONE',  ( 185.2500000000000000, 9.429780353434619030E-16, -7.700000000000000178 ) ) ;
#81214=ORIENTED_EDGE ( 'NONE', *, *, #25458, .T. ) ;
#81308=CARTESIAN_POINT ( 'NONE',  ( 187.4218750003414016, 0.000000000000000000, 7.564683531250000925 ) ) ;
#81315=CARTESIAN_POINT ( 'NONE',  ( 187.5000000000000000, 0.000000000000000000, 0.000000000000000000 ) ) ;
#81403=CARTESIAN_POINT ( 'NONE',  ( 184.6093750003413732, 9.264065473108010111E-16, -7.564683531250000925 ) ) ;
#81411=CARTESIAN_POINT ( 'NONE',  ( 185.1718750003414016, 9.264065473108010111E-16, -7.564683531250000925 ) ) ;
#81551=CARTESIAN_POINT ( 'NONE',  ( 187.2760416670080588, 6.551208109652274736, 3.782341765625001351 ) ) ;
#81604=CARTESIAN_POINT ( 'NONE',  ( 187.0677083336747444, -4.367472073101514418, -7.564683531250002702 ) ) ;
#81638=DIRECTION ( 'NONE',  ( 0.4999999999999471534, 0.000000000000000000, 0.8660254037844692387 ) ) ;
#81709=CARTESIAN_POINT ( 'NONE',  ( 184.5000000000000000, 9.429780353434619030E-16, 7.699999999999999289 ) ) ;
#81774=CARTESIAN_POINT ( 'NONE',  ( 184.0833333333333144, -6.668395609140180369, 3.849999999999994760 ) ) ;
#82024=CARTESIAN_POINT ( 'NONE',  ( 184.1510416670080588, 4.367472073101518859, -7.564683531249999149 ) ) ;
#82080=CARTESIAN_POINT ( 'NONE',  ( 195.5000000000000000, 6.123233995736766282E-16, 5.000000000000000000 ) ) ;
#82135=VERTEX_POINT ( 'NONE', #11175 ) ;
#82199=CARTESIAN_POINT ( 'NONE',  ( 187.3177083336747444, 4.367472073101515306, 7.564683531250000925 ) ) ;
#82264=CARTESIAN_POINT ( 'NONE',  ( 185.1562500006828031, 8.891194145520236347, 5.444286225454521982E-16 ) ) ;
#82540=VERTEX_POINT ( 'NONE', #49047 ) ;
#82563=CARTESIAN_POINT ( 'NONE',  ( 184.5000000000000284, -7.608433918590866263, 0.5575073813830642155 ) ) ;
#82600=CARTESIAN_POINT ( 'NONE',  ( 187.2135416670080588, 4.367472073101518859, -7.564683531249999149 ) ) ;
#82602=CARTESIAN_POINT ( 'NONE',  ( 186.5885416670080872, -6.551208109652273848, -3.782341765625003571 ) ) ;
#82634=DIRECTION ( 'NONE',  ( -1.000000000000000000, 0.000000000000000000, 0.000000000000000000 ) ) ;
#82700=( BOUNDED_CURVE ( )  B_SPLINE_CURVE ( 2, ( #102418, #91950, #12722, #82792, #112882, #42214, #123972 ),
 .UNSPECIFIED., .F., .F. ) 
 B_SPLINE_CURVE_WITH_KNOTS ( ( 3, 2, 2, 3 ),
 ( 0.5714285714285719520, 0.5952380952380957879, 0.6190476190476195129, 0.6428571428571433488 ),
 .UNSPECIFIED. ) 
 CURVE ( )  GEOMETRIC_REPRESENTATION_ITEM ( )  RATIONAL_B_SPLINE_CURVE ( ( 0.9999999999999968914, 0.8660254037844418162, 1.000000000000000000, 0.8660254037844387076, 1.000000000000000000, 0.8660254037844361541, 1.000000000000002442 ) ) 
 REPRESENTATION_ITEM ( '' )  );
#82778=ORIENTED_EDGE ( 'NONE', *, *, #84262, .F. ) ;
#82792=CARTESIAN_POINT ( 'NONE',  ( 185.3750000000000000, 8.891194145520236347, 5.444286225454521982E-16 ) ) ;
#82858=CARTESIAN_POINT ( 'NONE',  ( 185.7760416670080588, 6.551208109652274736, 3.782341765625001351 ) ) ;
#82908=CARTESIAN_POINT ( 'NONE',  ( 184.9479166673494603, -6.668395609140176816, -3.850000000000003642 ) ) ;
#82972=ORIENTED_EDGE ( 'NONE', *, *, #39529, .T. ) ;
#83112=DIRECTION ( 'NONE',  ( 1.000000000000000000, 0.000000000000000000, 0.000000000000000000 ) ) ;
#83245=CARTESIAN_POINT ( 'NONE',  ( 184.6718750003414016, 9.264065473108010111E-16, -7.564683531250000925 ) ) ;
#83260=CARTESIAN_POINT ( 'NONE',  ( 187.4166666666666856, 6.668395609140176816, 3.850000000000000977 ) ) ;
#83499=CARTESIAN_POINT ( 'NONE',  ( 185.1093750003413732, 9.264065473108010111E-16, -7.564683531250000925 ) ) ;
#83555=CARTESIAN_POINT ( 'NONE',  ( 183.7812500006828031, 0.000000000000000000, 7.700000000000000178 ) ) ;
#83687=DIRECTION ( 'NONE',  ( -0.9961946980917455452, 0.000000000000000000, -0.08715574274765836016 ) ) ;
#83766=CIRCLE ( 'NONE', #73294, 8.699999999999999289 ) ;
#83816=CARTESIAN_POINT ( 'NONE',  ( 194.5000000000000000, 4.898587196589412829E-16, 4.000000000000000000 ) ) ;
#83836=DIRECTION ( 'NONE',  ( 1.000000000000000000, -0.000000000000000000, -0.000000000000000000 ) ) ;
#83864=CARTESIAN_POINT ( 'NONE',  ( 186.5468750003414300, -8.734944146203032389, -1.604583208406768146E-15 ) ) ;
#83867=CARTESIAN_POINT ( 'NONE',  ( 186.9635416670080303, -4.367472073101520635, 7.564683531249999149 ) ) ;
#83897=CARTESIAN_POINT ( 'NONE',  ( 187.2760416670080588, 6.551208109652274736, 3.782341765625001351 ) ) ;
#83957=DIRECTION ( 'NONE',  ( 0.000000000000000000, 0.000000000000000000, 1.000000000000000000 ) ) ;
#84117=CARTESIAN_POINT ( 'NONE',  ( 185.9010416670080303, -4.367472073101519747, 7.564683531249999149 ) ) ;
#84134=DIRECTION ( 'NONE',  ( 1.000000000000000000, -0.000000000000000000, -0.000000000000000000 ) ) ;
#84172=CARTESIAN_POINT ( 'NONE',  ( 185.8177083336747444, 4.367472073101515306, 7.564683531250000925 ) ) ;
#84182=AXIS2_PLACEMENT_3D ( 'NONE', #75896, #74614, #25494 ) ;
#84232=CARTESIAN_POINT ( 'NONE',  ( 184.5000000000000284, -3.559465329748744633, -6.843514285309209022 ) ) ;
#84262=EDGE_CURVE ( 'NONE', #27061, #54972, #65650, .T. ) ;
#84395=DIRECTION ( 'NONE',  ( 1.000000000000000000, -0.000000000000000000, -0.000000000000000000 ) ) ;
#84500=DIRECTION ( 'NONE',  ( 0.000000000000000000, 0.000000000000000000, -1.000000000000000000 ) ) ;
#84520=CARTESIAN_POINT ( 'NONE',  ( 186.3385416670080872, 6.551208109652274736, 3.782341765625001351 ) ) ;
#84661=CARTESIAN_POINT ( 'NONE',  ( 185.5312500006828031, 9.429780353434619030E-16, -7.700000000000000178 ) ) ;
#84717=ORIENTED_EDGE ( 'NONE', *, *, #72761, .F. ) ;
#84774=CARTESIAN_POINT ( 'NONE',  ( 184.4010416670080872, -4.367472073101519747, 7.564683531249999149 ) ) ;
#84787=EDGE_LOOP ( 'NONE', ( #86146, #86501, #122878, #43196 ) ) ;
#84821=CARTESIAN_POINT ( 'NONE',  ( 185.3593750003413732, 0.000000000000000000, 7.564683531250000925 ) ) ;
#84829=CARTESIAN_POINT ( 'NONE',  ( 194.5000000000000000, 0.000000000000000000, 0.000000000000000000 ) ) ;
#84842=DIRECTION ( 'NONE',  ( 0.000000000000000000, 0.000000000000000000, 1.000000000000000000 ) ) ;
#85162=CARTESIAN_POINT ( 'NONE',  ( 185.3802083336747160, 4.367472073101515306, 7.564683531250000925 ) ) ;
#85164=CARTESIAN_POINT ( 'NONE',  ( 185.1718750003414016, 9.264065473108010111E-16, -7.564683531250000925 ) ) ;
#85328=ADVANCED_FACE ( 'NONE', ( #88939 ), #8425, .T. ) ;
#85379=EDGE_CURVE ( 'NONE', #120770, #82540, #73491, .T. ) ;
#85389=DIRECTION ( 'NONE',  ( -1.000000000000000000, 0.000000000000000000, 0.000000000000000000 ) ) ;
#85413=CARTESIAN_POINT ( 'NONE',  ( 185.3385416670080872, 6.551208109652274736, 3.782341765625001351 ) ) ;
#85469=CARTESIAN_POINT ( 'NONE',  ( 184.9010416670080588, -4.367472073101519747, 7.564683531249999149 ) ) ;
#85558=CARTESIAN_POINT ( 'NONE',  ( 194.5000000000000000, 0.000000000000000000, -4.000000000000000000 ) ) ;
#85590=VERTEX_POINT ( 'NONE', #12926 ) ;
#85797=CARTESIAN_POINT ( 'NONE',  ( 186.7135416670080872, 4.367472073101518859, -7.564683531249999149 ) ) ;
#85800=CARTESIAN_POINT ( 'NONE',  ( 184.8802083336747444, 4.367472073101515306, 7.564683531250000925 ) ) ;
#85827=CARTESIAN_POINT ( 'NONE',  ( 186.4843750003414016, -8.734944146203032389, -1.604583208406767949E-15 ) ) ;
#86035=CARTESIAN_POINT ( 'NONE',  ( 186.4218750003414016, 0.000000000000000000, 7.564683531250000925 ) ) ;
#86092=CARTESIAN_POINT ( 'NONE',  ( 186.3177083336747160, 4.367472073101515306, 7.564683531250000925 ) ) ;
#86111=ORIENTED_EDGE ( 'NONE', *, *, #69291, .T. ) ;
#86146=ORIENTED_EDGE ( 'NONE', *, *, #114868, .F. ) ;
#86336=CARTESIAN_POINT ( 'NONE',  ( 187.5000000000000000, 0.000000000000000000, 0.000000000000000000 ) ) ;
#86442=CARTESIAN_POINT ( 'NONE',  ( 184.1718750003414016, 9.264065473108010111E-16, -7.564683531250000925 ) ) ;
#86445=CARTESIAN_POINT ( 'NONE',  ( 185.5885416670080872, -6.551208109652273848, -3.782341765625003571 ) ) ;
#86478=CARTESIAN_POINT ( 'NONE',  ( 186.2343750003414016, 8.734944146203032389, 5.348610694689227483E-16 ) ) ;
#86499=VERTEX_POINT ( 'NONE', #126309 ) ;
#86501=ORIENTED_EDGE ( 'NONE', *, *, #25303, .F. ) ;
#86610=AXIS2_PLACEMENT_3D ( 'NONE', #549, #21492, #119681 ) ;
#86616=ORIENTED_EDGE ( 'NONE', *, *, #94769, .T. ) ;
#86703=CARTESIAN_POINT ( 'NONE',  ( 184.0260416670080588, -6.551208109652273848, -3.782341765625003571 ) ) ;
#86876=( BOUNDED_SURFACE ( )  B_SPLINE_SURFACE ( 1, 2, ( 
 ( #67917, #107847, #69862, #49591, #39777, #50232, #18170, #60696, #447, #29941, #109785, #117639, #79050, #68558, #58116, #58753, #100591, #98021, #20115, #48941, #60062, #80331, #88851, #120256, #90118, #39142, #99967, #70496, #118953, #29300, #110420, #12210, #90781, #50865, #62628, #23985, #22707, #3058, #101248, #43006, #23316, #43636, #122827, #32533, #53451, #1108, #71797, #92061, #101898, #120883, #63904, #82264, #63254, #103183, #41067, #91428, #82908, #121512, #21392, #13496, #113647, #10901, #111715, #93365, #61332, #102531, #72441, #52152, #33173, #3688, #12837, #52788, #80971, #122188, #42333, #112366, #92722, #73078, #11573, #2375, #22062, #113000, #31236, #51515, #83555 ),
 ( #123453, #33793, #73705, #71137, #111041, #1745, #41703, #81604, #31870, #61980, #34457, #25243, #126027, #6242, #54083, #44915, #46190, #124103, #5599, #44248, #66469, #74366, #14141, #94004, #4305, #86092, #55373, #114283, #95938, #94635, #65821, #65162, #64538, #36393, #35105, #76303, #105098, #84172, #125401, #116209, #26558, #56000, #4962, #106396, #24628, #104464, #14765, #54704, #84821, #15423, #16705, #124755, #25915, #95298, #75015, #115554, #114918, #45564, #75634, #85469, #105763, #16063, #103832, #35731, #74149, #91859, #81403, #123873, #31647, #34244, #2828, #13276, #72860, #2172, #114072, #102324, #63691, #82024, #12635, #102951, #24402, #112144, #112790, #51939, #52566 ) ),
 .UNSPECIFIED., .F., .F., .F. ) 
 B_SPLINE_SURFACE_WITH_KNOTS ( ( 2, 2 ),
 ( 3, 2, 2, 2, 2, 2, 2, 2, 2, 2, 2, 2, 2, 2, 2, 2, 2, 2, 2, 2, 2, 2, 2, 2, 2, 2, 2, 2, 2, 2, 2, 2, 2, 2, 2, 2, 2, 2, 2, 2, 2, 2, 3 ),
 ( 0.000000000000000000, 1.000000000000000000 ),
 ( 0.000000000000000000, 0.02380952380952380820, 0.04761904761904761640, 0.07142857142857142461, 0.09523809523809523281, 0.1190476190476190410, 0.1428571428571428492, 0.1666666666666666574, 0.1904761904761904656, 0.2142857142857142738, 0.2380952380952380820, 0.2619047619047619180, 0.2857142857142856984, 0.3095238095238095344, 0.3333333333333333148, 0.3571428571428571508, 0.3809523809523809312, 0.4047619047619047672, 0.4285714285714285476, 0.4523809523809523836, 0.4761904761904761640, 0.5000000000000000000, 0.5238095238095238360, 0.5476190476190476719, 0.5714285714285713969, 0.5952380952380952328, 0.6190476190476190688, 0.6428571428571429047, 0.6666666666666666297, 0.6904761904761904656, 0.7142857142857143016, 0.7380952380952381375, 0.7619047619047618625, 0.7857142857142856984, 0.8095238095238095344, 0.8333333333333333703, 0.8571428571428570953, 0.8809523809523809312, 0.9047619047619047672, 0.9285714285714286031, 0.9523809523809523281, 0.9761904761904761640, 1.000000000000000000 ),
 .UNSPECIFIED. ) 
 GEOMETRIC_REPRESENTATION_ITEM ( )  RATIONAL_B_SPLINE_SURFACE ( (
 ( 1.000000000000000000, 0.8660254037844387076, 1.000000000000000000, 0.8660254037844387076, 1.000000000000000000, 0.8660254037844387076, 1.000000000000000000, 0.8660254037844387076, 1.000000000000000000, 0.8660254037844387076, 1.000000000000000000, 0.8660254037844387076, 1.000000000000000000, 0.8660254037844387076, 1.000000000000000000, 0.8660254037844387076, 1.000000000000000000, 0.8660254037844387076, 1.000000000000000000, 0.8660254037844387076, 1.000000000000000000, 0.8660254037844387076, 1.000000000000000000, 0.8660254037844387076, 1.000000000000000000, 0.8660254037844387076, 1.000000000000000000, 0.8660254037844387076, 1.000000000000000000, 0.8660254037844387076, 1.000000000000000000, 0.8660254037844387076, 1.000000000000000000, 0.8660254037844387076, 1.000000000000000000, 0.8660254037844387076, 1.000000000000000000, 0.8660254037844387076, 1.000000000000000000, 0.8660254037844387076, 1.000000000000000000, 0.8660254037844387076, 1.000000000000000000, 0.8660254037844387076, 1.000000000000000000, 0.8660254037844387076, 1.000000000000000000, 0.8660254037844387076, 1.000000000000000000, 0.8660254037844387076, 1.000000000000000000, 0.8660254037844387076, 1.000000000000000000, 0.8660254037844387076, 1.000000000000000000, 0.8660254037844387076, 1.000000000000000000, 0.8660254037844387076, 1.000000000000000000, 0.8660254037844387076, 1.000000000000000000, 0.8660254037844387076, 1.000000000000000000, 0.8660254037844387076, 1.000000000000000000, 0.8660254037844387076, 1.000000000000000000, 0.8660254037844387076, 1.000000000000000000, 0.8660254037844387076, 1.000000000000000000, 0.8660254037844387076, 1.000000000000000000, 0.8660254037844387076, 1.000000000000000000, 0.8660254037844387076, 1.000000000000000000, 0.8660254037844387076, 1.000000000000000000, 0.8660254037844387076, 1.000000000000000000, 0.8660254037844387076, 1.000000000000000000, 0.8660254037844387076, 1.000000000000000000),
 ( 1.000000000000000000, 0.8660254037844387076, 1.000000000000000000, 0.8660254037844387076, 1.000000000000000000, 0.8660254037844387076, 1.000000000000000000, 0.8660254037844387076, 1.000000000000000000, 0.8660254037844387076, 1.000000000000000000, 0.8660254037844387076, 1.000000000000000000, 0.8660254037844387076, 1.000000000000000000, 0.8660254037844387076, 1.000000000000000000, 0.8660254037844387076, 1.000000000000000000, 0.8660254037844387076, 1.000000000000000000, 0.8660254037844387076, 1.000000000000000000, 0.8660254037844387076, 1.000000000000000000, 0.8660254037844387076, 1.000000000000000000, 0.8660254037844387076, 1.000000000000000000, 0.8660254037844387076, 1.000000000000000000, 0.8660254037844387076, 1.000000000000000000, 0.8660254037844387076, 1.000000000000000000, 0.8660254037844387076, 1.000000000000000000, 0.8660254037844387076, 1.000000000000000000, 0.8660254037844387076, 1.000000000000000000, 0.8660254037844387076, 1.000000000000000000, 0.8660254037844387076, 1.000000000000000000, 0.8660254037844387076, 1.000000000000000000, 0.8660254037844387076, 1.000000000000000000, 0.8660254037844387076, 1.000000000000000000, 0.8660254037844387076, 1.000000000000000000, 0.8660254037844387076, 1.000000000000000000, 0.8660254037844387076, 1.000000000000000000, 0.8660254037844387076, 1.000000000000000000, 0.8660254037844387076, 1.000000000000000000, 0.8660254037844387076, 1.000000000000000000, 0.8660254037844387076, 1.000000000000000000, 0.8660254037844387076, 1.000000000000000000, 0.8660254037844387076, 1.000000000000000000, 0.8660254037844387076, 1.000000000000000000, 0.8660254037844387076, 1.000000000000000000, 0.8660254037844387076, 1.000000000000000000, 0.8660254037844387076, 1.000000000000000000, 0.8660254037844387076, 1.000000000000000000, 0.8660254037844387076, 1.000000000000000000, 0.8660254037844387076, 1.000000000000000000, 0.8660254037844387076, 1.000000000000000000) ) ) 
 REPRESENTATION_ITEM ( '' )  SURFACE ( )  );
#87000=EDGE_LOOP ( 'NONE', ( #109544, #121824, #75068 ) ) ;
#87085=CARTESIAN_POINT ( 'NONE',  ( 186.5000000000000000, 0.000000000000000000, 7.700000000000000178 ) ) ;
#87166=ORIENTED_EDGE ( 'NONE', *, *, #80341, .F. ) ;
#87180=CIRCLE ( 'NONE', #105974, 5.000000000000000000 ) ;
#87211=FACE_BOUND ( 'NONE', #126452, .T. ) ;
#87284=EDGE_LOOP ( 'NONE', ( #88970, #80395, #97265, #77241 ) ) ;
#87331=CARTESIAN_POINT ( 'NONE',  ( 186.0468750003414300, -8.734944146203032389, -1.604583208406768146E-15 ) ) ;
#87392=PLANE ( 'NONE',  #3067 ) ;
#87423=CARTESIAN_POINT ( 'NONE',  ( 184.4999999999999716, -5.927738724303143414, 4.757631484588563886 ) ) ;
#87604=VERTEX_POINT ( 'NONE', #119039 ) ;
#87632=CARTESIAN_POINT ( 'NONE',  ( 184.7395833340161175, 4.445597072760175905, 7.699999999999896261 ) ) ;
#87643=DIRECTION ( 'NONE',  ( 1.000000000000000000, 0.000000000000000000, 0.000000000000000000 ) ) ;
#87729=CARTESIAN_POINT ( 'NONE',  ( 187.5000000000000000, 0.000000000000000000, 7.700000000000000178 ) ) ;
#87967=CARTESIAN_POINT ( 'NONE',  ( 185.3802083336747160, 4.367472073101515306, 7.564683531250000925 ) ) ;
#87978=EDGE_CURVE ( 'NONE', #85590, #17533, #32635, .T. ) ;
#87993=( LENGTH_UNIT ( ) NAMED_UNIT ( * ) SI_UNIT ( .MILLI., .METRE. ) );
#88084=CARTESIAN_POINT ( 'NONE',  ( 184.9062500006828031, -8.891194145520236347, -1.633285867636356299E-15 ) ) ;
#88264=DIRECTION ( 'NONE',  ( 1.000000000000000000, -0.000000000000000000, -0.000000000000000000 ) ) ;
#88365=CARTESIAN_POINT ( 'NONE',  ( 186.3333333333333144, 6.668395609140177704, -3.849999999999998312 ) ) ;
#88483=VECTOR ( 'NONE', #6511, 1000.000000000000000 ) ;
#88763=CARTESIAN_POINT ( 'NONE',  ( 184.8229166673494888, -4.445597072760063107, 7.700000000000102318 ) ) ;
#88851=CARTESIAN_POINT ( 'NONE',  ( 186.3645833340161175, -6.668395609140180369, 3.849999999999994760 ) ) ;
#88925=DIRECTION ( 'NONE',  ( 1.000000000000000000, -0.000000000000000000, -0.000000000000000000 ) ) ;
#88939=FACE_OUTER_BOUND ( 'NONE', #13972, .T. ) ;
#88970=ORIENTED_EDGE ( 'NONE', *, *, #68637, .F. ) ;
#88971=DIRECTION ( 'NONE',  ( -1.000000000000000000, 0.000000000000000000, 0.000000000000000000 ) ) ;
#89038=CARTESIAN_POINT ( 'NONE',  ( 184.8750000000000000, 8.891194145520236347, 5.444286225454521982E-16 ) ) ;
#89071=CARTESIAN_POINT ( 'NONE',  ( 185.6093750003413732, 9.264065473108010111E-16, -7.564683531250000925 ) ) ;
#89285=CARTESIAN_POINT ( 'NONE',  ( 184.1718750003414016, 9.264065473108010111E-16, -7.564683531250000925 ) ) ;
#89289=DIRECTION ( 'NONE',  ( -1.000000000000000000, -0.000000000000000000, -0.000000000000000000 ) ) ;
#89298=DIRECTION ( 'NONE',  ( 0.000000000000000000, 0.000000000000000000, -1.000000000000000000 ) ) ;
#89351=STYLED_ITEM ( 'NONE', ( #9462 ), #12695 ) ;
#89552=FACE_OUTER_BOUND ( 'NONE', #87000, .T. ) ;
#89668=ORIENTED_EDGE ( 'NONE', *, *, #110172, .F. ) ;
#89679=CARTESIAN_POINT ( 'NONE',  ( 184.0000000000000000, 0.000000000000000000, 7.700000000000000178 ) ) ;
#89706=CARTESIAN_POINT ( 'NONE',  ( 185.2760416670080588, 6.551208109652274736, 3.782341765625001351 ) ) ;
#89744=CARTESIAN_POINT ( 'NONE',  ( 187.0312500006828031, 9.429780353434619030E-16, -7.700000000000000178 ) ) ;
#89919=CARTESIAN_POINT ( 'NONE',  ( 184.9218750003414016, 0.000000000000000000, 7.564683531250000925 ) ) ;
#89975=FACE_OUTER_BOUND ( 'NONE', #107912, .T. ) ;
#90097=FACE_OUTER_BOUND ( 'NONE', #49095, .T. ) ;
#90118=CARTESIAN_POINT ( 'NONE',  ( 186.2812500006828031, 0.000000000000000000, 7.700000000000000178 ) ) ;
#90243=ORIENTED_EDGE ( 'NONE', *, *, #23726, .F. ) ;
#90360=CIRCLE ( 'NONE', #15125, 4.000000000000000000 ) ;
#90508=ORIENTED_EDGE ( 'NONE', *, *, #26068, .T. ) ;
#90516=DIRECTION ( 'NONE',  ( 0.000000000000000000, 0.000000000000000000, 1.000000000000000000 ) ) ;
#90578=DIRECTION ( 'NONE',  ( 0.000000000000000000, 0.000000000000000000, -1.000000000000000000 ) ) ;
#90663=ORIENTED_EDGE ( 'NONE', *, *, #67561, .F. ) ;
#90781=CARTESIAN_POINT ( 'NONE',  ( 185.9479166673494603, -6.668395609140176816, -3.850000000000003642 ) ) ;
#90784=VECTOR ( 'NONE', #7213, 1000.000000000000000 ) ;
#90960=FACE_OUTER_BOUND ( 'NONE', #108770, .T. ) ;
#90969=CARTESIAN_POINT ( 'NONE',  ( 185.0833333333333144, -6.668395609140180369, 3.849999999999994760 ) ) ;
#91083=( BOUNDED_CURVE ( )  B_SPLINE_CURVE ( 2, ( #56259, #126299, #47108, #28096, #27433, #58222, #36649 ),
 .UNSPECIFIED., .F., .F. ) 
 B_SPLINE_CURVE_WITH_KNOTS ( ( 3, 2, 2, 3 ),
 ( 0.6428571428571433488, 0.6666666666666670737, 0.6904761904761910207, 0.7142857142857148567 ),
 .UNSPECIFIED. ) 
 CURVE ( )  GEOMETRIC_REPRESENTATION_ITEM ( )  RATIONAL_B_SPLINE_CURVE ( ( 0.9999999999999974465, 0.8660254037844412611, 1.000000000000000000, 0.8660254037844387076, 1.000000000000000000, 0.8660254037844355990, 1.000000000000003109 ) ) 
 REPRESENTATION_ITEM ( '' )  );
#91123=CARTESIAN_POINT ( 'NONE',  ( 186.8802083336747444, 4.367472073101515306, 7.564683531250000925 ) ) ;
#91219=CARTESIAN_POINT ( 'NONE',  ( 184.7552083336747444, 6.551208109652275624, -3.782341765624998686 ) ) ;
#91300=CARTESIAN_POINT ( 'NONE',  ( 184.4999999999999716, -1.540470907863150662, 7.523675357873957914 ) ) ;
#91320=CARTESIAN_POINT ( 'NONE',  ( 185.7500000000000000, 9.429780353434619030E-16, -7.700000000000000178 ) ) ;
#91428=CARTESIAN_POINT ( 'NONE',  ( 184.9895833340161175, -4.445597072760115509, -7.700000000000001954 ) ) ;
#91609=CARTESIAN_POINT ( 'NONE',  ( 185.1250000000000284, -8.891194145520236347, -1.633285867636356693E-15 ) ) ;
#91613=VERTEX_POINT ( 'NONE', #97003 ) ;
#91752=PLANE ( 'NONE',  #18157 ) ;
#91762=CARTESIAN_POINT ( 'NONE',  ( 186.7552083336747444, 6.551208109652275624, -3.782341765624998686 ) ) ;
#91829=ORIENTED_EDGE ( 'NONE', *, *, #39988, .F. ) ;
#91846=EDGE_CURVE ( 'NONE', #100903, #65296, #83766, .T. ) ;
#91859=CARTESIAN_POINT ( 'NONE',  ( 184.6510416670080588, 4.367472073101518859, -7.564683531249999149 ) ) ;
#91863=( BOUNDED_CURVE ( )  B_SPLINE_CURVE ( 2, ( #57201, #76850, #107593, #6778, #116753, #27102, #127244 ),
 .UNSPECIFIED., .F., .F. ) 
 B_SPLINE_CURVE_WITH_KNOTS ( ( 3, 2, 2, 3 ),
 ( 0.000000000000000000, 0.02380952380952383249, 0.04761904761904766498, 0.07142857142857149400 ),
 .UNSPECIFIED. ) 
 CURVE ( )  GEOMETRIC_REPRESENTATION_ITEM ( )  RATIONAL_B_SPLINE_CURVE ( ( 1.000000000000000000, 0.8660254037844387076, 1.000000000000000000, 0.8660254037844387076, 1.000000000000000000, 0.8660254037844383745, 1.000000000000000444 ) ) 
 REPRESENTATION_ITEM ( '' )  );
#91950=CARTESIAN_POINT ( 'NONE',  ( 185.4583333333333428, 4.445597072760175905, 7.699999999999896261 ) ) ;
#92061=CARTESIAN_POINT ( 'NONE',  ( 185.3229166673494888, -4.445597072760122614, 7.699999999999998401 ) ) ;
#92084=DIRECTION ( 'NONE',  ( 1.000000000000000000, 0.000000000000000000, 0.000000000000000000 ) ) ;
#92155=ORIENTED_EDGE ( 'NONE', *, *, #91846, .T. ) ;
#92244=EDGE_CURVE ( 'NONE', #117178, #1307, #41818, .T. ) ;
#92314=CARTESIAN_POINT ( 'NONE',  ( 186.6666666666666856, -6.668395609140176816, -3.850000000000003642 ) ) ;
#92363=CARTESIAN_POINT ( 'NONE',  ( 187.1249999999999716, -8.891194145520236347, -1.633285867636356299E-15 ) ) ;
#92414=EDGE_LOOP ( 'NONE', ( #105031, #128574, #21121, #539 ) ) ;
#92556=ORIENTED_EDGE ( 'NONE', *, *, #53104, .T. ) ;
#92584=CARTESIAN_POINT ( 'NONE',  ( 194.5000000000000000, 4.898587196589412829E-16, 4.000000000000000000 ) ) ;
#92658=CARTESIAN_POINT ( 'NONE',  ( 186.2760416670080588, 6.551208109652274736, 3.782341765625001351 ) ) ;
#92722=CARTESIAN_POINT ( 'NONE',  ( 184.1145833340161175, 6.668395609140177704, -3.849999999999998312 ) ) ;
#92938=ORIENTED_EDGE ( 'NONE', *, *, #85379, .T. ) ;
#93065=CARTESIAN_POINT ( 'NONE',  ( 185.1302083336747160, -4.367472073101514418, -7.564683531250002702 ) ) ;
#93068=CARTESIAN_POINT ( 'NONE',  ( 186.5052083336747444, -6.551208109652278289, 3.782341765624995134 ) ) ;
#93308=CARTESIAN_POINT ( 'NONE',  ( 185.4843750003414300, -8.734944146203032389, -1.604583208406768146E-15 ) ) ;
#93365=CARTESIAN_POINT ( 'NONE',  ( 184.6562500006828031, 8.891194145520236347, 5.444286225454521982E-16 ) ) ;
#93696=CARTESIAN_POINT ( 'NONE',  ( 184.7552083336747444, 6.551208109652275624, -3.782341765624998686 ) ) ;
#93734=CARTESIAN_POINT ( 'NONE',  ( 186.0260416670080588, -6.551208109652273848, -3.782341765625003571 ) ) ;
#93952=CARTESIAN_POINT ( 'NONE',  ( 195.5000000000000000, 0.000000000000000000, 0.000000000000000000 ) ) ;
#93953=CARTESIAN_POINT ( 'NONE',  ( 186.5677083336747160, -4.367472073101514418, -7.564683531250002702 ) ) ;
#94004=CARTESIAN_POINT ( 'NONE',  ( 186.4010416670080588, -4.367472073101519747, 7.564683531249999149 ) ) ;
#94054=CARTESIAN_POINT ( 'NONE',  ( 187.0000000000000000, 0.000000000000000000, 7.700000000000000178 ) ) ;
#94131=ORIENTED_EDGE ( 'NONE', *, *, #64227, .T. ) ;
#94190=VECTOR ( 'NONE', #44172, 1000.000000000000000 ) ;
#94191=ORIENTED_EDGE ( 'NONE', *, *, #38635, .T. ) ;
#94288=CARTESIAN_POINT ( 'NONE',  ( 184.5000000000000568, -7.615651362878065989, -0.4485267508106103307 ) ) ;
#94324=CARTESIAN_POINT ( 'NONE',  ( 187.1718750003414016, 9.264065473108010111E-16, -7.564683531250000925 ) ) ;
#94327=CARTESIAN_POINT ( 'NONE',  ( 185.2968750003414300, 8.734944146203032389, 5.348610694689227483E-16 ) ) ;
#94362=CARTESIAN_POINT ( 'NONE',  ( 185.8593750003413732, 0.000000000000000000, 7.564683531250000925 ) ) ;
#94452=CARTESIAN_POINT ( 'NONE',  ( 184.5000000000000000, 0.000000000000000000, -5.200000000000000178 ) ) ;
#94463=AXIS2_PLACEMENT_3D ( 'NONE', #7681, #74511, #47629 ) ;
#94464=CARTESIAN_POINT ( 'NONE',  ( 185.6979166673494603, 6.668395609140176816, 3.850000000000000977 ) ) ;
#94578=CARTESIAN_POINT ( 'NONE',  ( 185.4427083336747160, -6.551208109652278289, 3.782341765624995134 ) ) ;
#94635=CARTESIAN_POINT ( 'NONE',  ( 186.1510416670080588, 4.367472073101518859, -7.564683531249999149 ) ) ;
#94769=EDGE_CURVE ( 'NONE', #70723, #26135, #48602, .T. ) ;
#94833=CARTESIAN_POINT ( 'NONE',  ( 184.5000000000000000, 0.000000000000000000, 0.000000000000000000 ) ) ;
#94924=ORIENTED_EDGE ( 'NONE', *, *, #41000, .F. ) ;
#94993=CARTESIAN_POINT ( 'NONE',  ( 186.1302083336747444, -4.367472073101514418, -7.564683531250002702 ) ) ;
#95028=CARTESIAN_POINT ( 'NONE',  ( 186.9010416670080588, -4.367472073101520635, 7.564683531249999149 ) ) ;
#95223=CIRCLE ( 'NONE', #9449, 7.541925104783893552 ) ;
#95244=CARTESIAN_POINT ( 'NONE',  ( 184.9843750003414016, -8.734944146203032389, -1.604583208406768146E-15 ) ) ;
#95250=EDGE_CURVE ( 'NONE', #39170, #82540, #117805, .T. ) ;
#95294=( BOUNDED_CURVE ( )  B_SPLINE_CURVE ( 2, ( #89744, #109381, #50457, #110038, #119847, #712, #60310 ),
 .UNSPECIFIED., .F., .F. ) 
 B_SPLINE_CURVE_WITH_KNOTS ( ( 3, 2, 2, 3 ),
 ( 0.07142857142857149400, 0.09523809523809532995, 0.1190476190476191520, 0.1428571428571429880 ),
 .UNSPECIFIED. ) 
 CURVE ( )  GEOMETRIC_REPRESENTATION_ITEM ( )  RATIONAL_B_SPLINE_CURVE ( ( 0.9999999999999996669, 0.8660254037844390407, 1.000000000000000000, 0.8660254037844387076, 1.000000000000000000, 0.8660254037844379305, 1.000000000000000666 ) ) 
 REPRESENTATION_ITEM ( '' )  );
#95298=CARTESIAN_POINT ( 'NONE',  ( 185.1510416670080872, 4.367472073101518859, -7.564683531249999149 ) ) ;
#95322=DIRECTION ( 'NONE',  ( -1.000000000000000000, 0.000000000000000000, 0.000000000000000000 ) ) ;
#95606=MECHANICAL_DESIGN_GEOMETRIC_PRESENTATION_REPRESENTATION('',(#89351),#110273);
#95633=CARTESIAN_POINT ( 'NONE',  ( 184.8802083336747444, 4.367472073101515306, 7.564683531250000925 ) ) ;
#95635=CARTESIAN_POINT ( 'NONE',  ( 185.9635416670080588, -4.367472073101520635, 7.564683531249999149 ) ) ;
#95645=CARTESIAN_POINT ( 'NONE',  ( 187.5000000000000000, 0.000000000000000000, 7.700000000000000178 ) ) ;
#95885=CARTESIAN_POINT ( 'NONE',  ( 186.7552083336747444, 6.551208109652275624, -3.782341765624998686 ) ) ;
#95909=CARTESIAN_POINT ( 'NONE',  ( 184.5000000000000000, 0.000000000000000000, 0.000000000000000000 ) ) ;
#95938=CARTESIAN_POINT ( 'NONE',  ( 186.1927083336747160, 6.551208109652275624, -3.782341765624998686 ) ) ;
#95969=CARTESIAN_POINT ( 'NONE',  ( 184.5000000000000000, 0.000000000000000000, -7.699999999999999289 ) ) ;
#96054=( BOUNDED_CURVE ( )  B_SPLINE_CURVE ( 2, ( #110203, #72854, #13270, #53224, #3467, #123246, #35516 ),
 .UNSPECIFIED., .F., .F. ) 
 B_SPLINE_CURVE_WITH_KNOTS ( ( 3, 2, 2, 3 ),
 ( 0.7142857142857148567, 0.7380952380952386926, 0.7619047619047624176, 0.7857142857142862535 ),
 .UNSPECIFIED. ) 
 CURVE ( )  GEOMETRIC_REPRESENTATION_ITEM ( )  RATIONAL_B_SPLINE_CURVE ( ( 0.9999999999999968914, 0.8660254037844418162, 1.000000000000000000, 0.8660254037844387076, 1.000000000000000000, 0.8660254037844355990, 1.000000000000003109 ) ) 
 REPRESENTATION_ITEM ( '' )  );
#96254=CARTESIAN_POINT ( 'NONE',  ( 183.9635416670080872, -4.367472073101519747, 7.564683531249999149 ) ) ;
#96256=CARTESIAN_POINT ( 'NONE',  ( 184.5026531346524905, -6.417290985200525100, 4.014293029178955585 ) ) ;
#96419=CARTESIAN_POINT ( 'NONE',  ( 185.1145833340161175, 6.668395609140177704, -3.849999999999998312 ) ) ;
#96500=CARTESIAN_POINT ( 'NONE',  ( 185.5885416670080872, -6.551208109652273848, -3.782341765625003571 ) ) ;
#96647=LINE ( 'NONE', #85558, #49959 ) ;
#96789=ORIENTED_EDGE ( 'NONE', *, *, #99642, .F. ) ;
#96844=DIRECTION ( 'NONE',  ( 1.000000000000000000, -0.000000000000000000, -0.000000000000000000 ) ) ;
#96909=CARTESIAN_POINT ( 'NONE',  ( 184.5052083336747444, -6.551208109652278289, 3.782341765624995134 ) ) ;
#96912=CARTESIAN_POINT ( 'NONE',  ( 186.0468750003414300, -8.734944146203032389, -1.604583208406767949E-15 ) ) ;
#97003=CARTESIAN_POINT ( 'NONE',  ( 185.7812500006828031, 0.000000000000000000, 7.700000000000000178 ) ) ;
#97035=ORIENTED_EDGE ( 'NONE', *, *, #91846, .F. ) ;
#97050=DIRECTION ( 'NONE',  ( 0.000000000000000000, 1.224646799147355426E-16, 1.000000000000000000 ) ) ;
#97169=CARTESIAN_POINT ( 'NONE',  ( 185.2135416670080872, 4.367472073101518859, -7.564683531249999149 ) ) ;
#97220=VERTEX_POINT ( 'NONE', #94054 ) ;
#97265=ORIENTED_EDGE ( 'NONE', *, *, #68206, .F. ) ;
#97440=VERTEX_POINT ( 'NONE', #91320 ) ;
#97525=CARTESIAN_POINT ( 'NONE',  ( 186.1979166673494603, 6.668395609140176816, 3.850000000000000977 ) ) ;
#97557=CARTESIAN_POINT ( 'NONE',  ( 186.6666666666666856, -6.668395609140176816, -3.850000000000003642 ) ) ;
#97590=CARTESIAN_POINT ( 'NONE',  ( 185.6927083336747160, 6.551208109652275624, -3.782341765624998686 ) ) ;
#97684=ORIENTED_EDGE ( 'NONE', *, *, #65483, .T. ) ;
#97807=CARTESIAN_POINT ( 'NONE',  ( 187.3385416670080872, 6.551208109652274736, 3.782341765625001351 ) ) ;
#97890=CARTESIAN_POINT ( 'NONE',  ( 184.5000000000000000, -2.439371826966624468, 7.284141803326471099 ) ) ;
#97925=( GEOMETRIC_REPRESENTATION_CONTEXT ( 3 ) GLOBAL_UNCERTAINTY_ASSIGNED_CONTEXT ( ( #129187 ) ) GLOBAL_UNIT_ASSIGNED_CONTEXT ( ( #57700, #66852, #8563 ) ) REPRESENTATION_CONTEXT ( 'NONE', 'WORKASPACE' ) );
#98021=CARTESIAN_POINT ( 'NONE',  ( 186.5729166673494603, 4.445597072760120838, -7.699999999999998401 ) ) ;
#98041=PRODUCT_DEFINITION ( 'UNKNOWN', '', #69288, #36291 ) ;
#98052=CARTESIAN_POINT ( 'NONE',  ( 187.5000000000000000, -1.065442715258197248E-15, 8.699999999999999289 ) ) ;
#98056=AXIS2_PLACEMENT_3D ( 'NONE', #42874, #111582, #22582 ) ;
#98163=ORIENTED_EDGE ( 'NONE', *, *, #64374, .T. ) ;
#98201=CARTESIAN_POINT ( 'NONE',  ( 185.8333333333333144, 6.668395609140177704, -3.849999999999998312 ) ) ;
#98232=CARTESIAN_POINT ( 'NONE',  ( 185.1093750003413732, 9.264065473108010111E-16, -7.564683531250000925 ) ) ;
#98348=CARTESIAN_POINT ( 'NONE',  ( 185.5416666666666856, -4.445597072760063107, 7.700000000000102318 ) ) ;
#98440=CARTESIAN_POINT ( 'NONE',  ( 185.7552083336747444, 6.551208109652275624, -3.782341765624998686 ) ) ;
#98456=CARTESIAN_POINT ( 'NONE',  ( 194.5000000000000000, 0.000000000000000000, 0.000000000000000000 ) ) ;
#98472=EDGE_LOOP ( 'NONE', ( #128418, #40909 ) ) ;
#98842=CARTESIAN_POINT ( 'NONE',  ( 187.1250000000000284, -8.891194145520236347, -1.633285867636356693E-15 ) ) ;
#98877=CARTESIAN_POINT ( 'NONE',  ( 185.4427083336747160, -6.551208109652278289, 3.782341765624995134 ) ) ;
#99057=UNCERTAINTY_MEASURE_WITH_UNIT (LENGTH_MEASURE( 1.000000000000000082E-05 ), #67478, 'distance_accuracy_value', 'NONE');
#99113=CARTESIAN_POINT ( 'NONE',  ( 184.4635416670080588, -4.367472073101519747, 7.564683531249999149 ) ) ;
#99122=VERTEX_POINT ( 'NONE', #51922 ) ;
#99124=CARTESIAN_POINT ( 'NONE',  ( 187.5000000000000000, 0.000000000000000000, 7.700000000000000178 ) ) ;
#99255=CARTESIAN_POINT ( 'NONE',  ( 186.2916666666666288, 4.445597072760091528, -7.700000000000049916 ) ) ;
#99402=DIRECTION ( 'NONE',  ( 0.000000000000000000, 0.000000000000000000, -1.000000000000000000 ) ) ;
#99509=( BOUNDED_CURVE ( )  B_SPLINE_CURVE ( 2, ( #66890, #17116, #3634, #107472, #57741, #16493, #43584 ),
 .UNSPECIFIED., .F., .F. ) 
 B_SPLINE_CURVE_WITH_KNOTS ( ( 3, 2, 2, 3 ),
 ( 0.3571428571428574283, 0.3809523809523812643, 0.4047619047619051003, 0.4285714285714289362 ),
 .UNSPECIFIED. ) 
 CURVE ( )  GEOMETRIC_REPRESENTATION_ITEM ( )  RATIONAL_B_SPLINE_CURVE ( ( 0.9999999999999984457, 0.8660254037844402619, 1.000000000000000000, 0.8660254037844387076, 1.000000000000000000, 0.8660254037844364872, 1.000000000000002220 ) ) 
 REPRESENTATION_ITEM ( '' )  );
#99514=CARTESIAN_POINT ( 'NONE',  ( 184.0416666666666572, -4.445597072760122614, 7.699999999999998401 ) ) ;
#99642=EDGE_CURVE ( 'NONE', #99122, #34917, #96647, .T. ) ;
#99647=DIRECTION ( 'NONE',  ( -1.000000000000000000, 0.000000000000000000, 0.000000000000000000 ) ) ;
#99741=VERTEX_POINT ( 'NONE', #92584 ) ;
#99787=EDGE_LOOP ( 'NONE', ( #123935, #2714 ) ) ;
#99815=DIRECTION ( 'NONE',  ( 0.000000000000000000, 0.000000000000000000, -1.000000000000000000 ) ) ;
#99967=CARTESIAN_POINT ( 'NONE',  ( 186.1979166673494603, 6.668395609140176816, 3.850000000000000977 ) ) ;
#100034=LINE ( 'NONE', #48348, #106620 ) ;
#100041=CARTESIAN_POINT ( 'NONE',  ( 195.0000000000000000, 0.000000000000000000, 0.000000000000000000 ) ) ;
#100103=CIRCLE ( 'NONE', #43690, 7.699999999999999289 ) ;
#100130=CARTESIAN_POINT ( 'NONE',  ( 186.4895833340161460, -4.445597072760135937, -7.699999999999966427 ) ) ;
#100141=CARTESIAN_POINT ( 'NONE',  ( 195.0000000000000000, 0.000000000000000000, 0.000000000000000000 ) ) ;
#100260=ORIENTED_EDGE ( 'NONE', *, *, #16544, .T. ) ;
#100267=( BOUNDED_CURVE ( )  B_SPLINE_CURVE ( 2, ( #119003, #118353, #107890, #49640, #28703, #109166, #68606 ),
 .UNSPECIFIED., .F., .F. ) 
 B_SPLINE_CURVE_WITH_KNOTS ( ( 3, 2, 2, 3 ),
 ( 0.1428571428571429880, 0.1666666666666668239, 0.1904761904761906322, 0.2142857142857144681 ),
 .UNSPECIFIED. ) 
 CURVE ( )  GEOMETRIC_REPRESENTATION_ITEM ( )  RATIONAL_B_SPLINE_CURVE ( ( 0.9999999999999992228, 0.8660254037844394848, 1.000000000000000000, 0.8660254037844387076, 1.000000000000000000, 0.8660254037844375974, 1.000000000000001110 ) ) 
 REPRESENTATION_ITEM ( '' )  );
#100291=FACE_BOUND ( 'NONE', #56484, .T. ) ;
#100354=CARTESIAN_POINT ( 'NONE',  ( 185.9166666666666856, 6.668395609140176816, 3.850000000000000977 ) ) ;
#100360=ADVANCED_FACE ( 'NONE', ( #1685 ), #76180, .T. ) ;
#100432=ORIENTED_EDGE ( 'NONE', *, *, #73518, .F. ) ;
#100591=CARTESIAN_POINT ( 'NONE',  ( 186.6145833340161175, 6.668395609140177704, -3.849999999999998312 ) ) ;
#100880=FACE_OUTER_BOUND ( 'NONE', #113195, .T. ) ;
#100903=VERTEX_POINT ( 'NONE', #125505 ) ;
#101177=CARTESIAN_POINT ( 'NONE',  ( 186.2500000000000000, 9.429780353434619030E-16, -7.700000000000000178 ) ) ;
#101248=CARTESIAN_POINT ( 'NONE',  ( 185.6979166673494603, 6.668395609140176816, 3.850000000000000977 ) ) ;
#101433=CARTESIAN_POINT ( 'NONE',  ( 185.2916666666666572, 4.445597072760120838, -7.699999999999998401 ) ) ;
#101555=B_SPLINE_CURVE_WITH_KNOTS ( 'NONE', 3,
 ( #15054, #94288, #82563, #32186, #112015, #2677 ),
 .UNSPECIFIED., .F., .F.,
 ( 4, 2, 4 ),
 ( 0.000000000000000000, 0.002961986837177525006, 0.005923973674355050012 ),
 .UNSPECIFIED. ) ;
#101599=AXIS2_PLACEMENT_3D ( 'NONE', #103390, #83112, #125585 ) ;
#101654=ADVANCED_FACE ( 'NONE', ( #28460, #68362 ), #108290, .T. ) ;
#101705=CARTESIAN_POINT ( 'NONE',  ( 184.5000000000000000, 0.000000000000000000, 0.000000000000000000 ) ) ;
#101709=FACE_OUTER_BOUND ( 'NONE', #87284, .T. ) ;
#101886=VERTEX_POINT ( 'NONE', #34265 ) ;
#101898=CARTESIAN_POINT ( 'NONE',  ( 185.2812500006828031, 0.000000000000000000, 7.700000000000000178 ) ) ;
#101936=LINE ( 'NONE', #10328, #8935 ) ;
#102040=CARTESIAN_POINT ( 'NONE',  ( 184.5000000000000000, 0.000000000000000000, 7.700000000000000178 ) ) ;
#102140=STYLED_ITEM ( 'NONE', ( #47237 ), #25840 ) ;
#102227=EDGE_CURVE ( 'NONE', #54972, #55284, #101555, .T. ) ;
#102235=CARTESIAN_POINT ( 'NONE',  ( 187.3385416670080872, 6.551208109652274736, 3.782341765625001351 ) ) ;
#102289=CARTESIAN_POINT ( 'NONE',  ( 185.4479166673494603, -6.668395609140176816, -3.850000000000003642 ) ) ;
#102324=CARTESIAN_POINT ( 'NONE',  ( 184.2343750003414016, 8.734944146203032389, 5.348610694689227483E-16 ) ) ;
#102418=CARTESIAN_POINT ( 'NONE',  ( 185.5000000000000000, 0.000000000000000000, 7.700000000000000178 ) ) ;
#102478=CARTESIAN_POINT ( 'NONE',  ( 186.7760416670080588, 6.551208109652274736, 3.782341765625001351 ) ) ;
#102531=CARTESIAN_POINT ( 'NONE',  ( 184.5729166673494603, 4.445597072760120838, -7.699999999999998401 ) ) ;
#102701=LINE ( 'NONE', #637, #6886 ) ;
#102718=CYLINDRICAL_SURFACE ( 'NONE', #5433, 5.200000000000000178 ) ;
#102787=CIRCLE ( 'NONE', #17088, 7.699999999999999289 ) ;
#102853=CARTESIAN_POINT ( 'NONE',  ( 186.6718750003414016, 9.264065473108010111E-16, -7.564683531250000925 ) ) ;
#102855=CARTESIAN_POINT ( 'NONE',  ( 186.5468750003414300, -8.734944146203032389, -1.604583208406767949E-15 ) ) ;
#102875=AXIS2_PLACEMENT_3D ( 'NONE', #100041, #18885, #99402 ) ;
#102895=EDGE_CURVE ( 'NONE', #44517, #22601, #4558, .T. ) ;
#102951=CARTESIAN_POINT ( 'NONE',  ( 184.0677083336747160, -4.367472073101514418, -7.564683531250002702 ) ) ;
#102981=CARTESIAN_POINT ( 'NONE',  ( 195.0000000000000000, 0.000000000000000000, 0.000000000000000000 ) ) ;
#103121=CARTESIAN_POINT ( 'NONE',  ( 186.6927083336747160, 6.551208109652275624, -3.782341765624998686 ) ) ;
#103183=CARTESIAN_POINT ( 'NONE',  ( 185.0729166673494888, 4.445597072760120838, -7.699999999999998401 ) ) ;
#103324=CYLINDRICAL_SURFACE ( 'NONE', #60424, 7.699999999999999289 ) ;
#103386=ADVANCED_FACE ( 'NONE', ( #124367 ), #13742, .T. ) ;
#103390=CARTESIAN_POINT ( 'NONE',  ( 195.0000000000000000, 0.000000000000000000, 0.000000000000000000 ) ) ;
#103413=CIRCLE ( 'NONE', #28103, 0.4999999999999995559 ) ;
#103433=CARTESIAN_POINT ( 'NONE',  ( 185.0000000000000000, 0.000000000000000000, 7.700000000000000178 ) ) ;
#103522=CARTESIAN_POINT ( 'NONE',  ( 185.8385416670080872, 6.551208109652274736, 3.782341765625001351 ) ) ;
#103524=CARTESIAN_POINT ( 'NONE',  ( 186.2968750003414584, 8.734944146203032389, 5.348610694689227483E-16 ) ) ;
#103543=CARTESIAN_POINT ( 'NONE',  ( 187.3750000000000000, 8.891194145520236347, 5.444286225454521982E-16 ) ) ;
#103581=CARTESIAN_POINT ( 'NONE',  ( 186.7916666666667140, 4.445597072760099522, -7.700000000000035705 ) ) ;
#103775=CARTESIAN_POINT ( 'NONE',  ( 184.7343750003414016, 8.734944146203032389, 5.348610694689227483E-16 ) ) ;
#103788=EDGE_CURVE ( 'NONE', #34917, #44517, #2707, .T. ) ;
#103832=CARTESIAN_POINT ( 'NONE',  ( 184.7760416670080588, 6.551208109652274736, 3.782341765625001351 ) ) ;
#103904=ORIENTED_EDGE ( 'NONE', *, *, #49126, .F. ) ;
#103912=EDGE_CURVE ( 'NONE', #99741, #16266, #45202, .T. ) ;
#104079=CARTESIAN_POINT ( 'NONE',  ( 186.7083333333333428, -4.445597072760135937, -7.699999999999966427 ) ) ;
#104160=CARTESIAN_POINT ( 'NONE',  ( 186.5052083336747444, -6.551208109652278289, 3.782341765624995134 ) ) ;
#104244=CARTESIAN_POINT ( 'NONE',  ( 185.9062500006827747, -8.891194145520236347, -1.633285867636356299E-15 ) ) ;
#104291=CARTESIAN_POINT ( 'NONE',  ( 195.5000000000000000, 9.541191101069066007E-16, 7.541925104783893552 ) ) ;
#104412=CARTESIAN_POINT ( 'NONE',  ( 184.5260416670080588, -6.551208109652273848, -3.782341765625003571 ) ) ;
#104464=CARTESIAN_POINT ( 'NONE',  ( 185.4843750003414300, -8.734944146203032389, -1.604583208406768146E-15 ) ) ;
#104470=DIRECTION ( 'NONE',  ( 0.000000000000000000, 0.000000000000000000, -1.000000000000000000 ) ) ;
#104712=ORIENTED_EDGE ( 'NONE', *, *, #40311, .F. ) ;
#104782=CARTESIAN_POINT ( 'NONE',  ( 186.9635416670080303, -4.367472073101519747, 7.564683531249999149 ) ) ;
#104784=CARTESIAN_POINT ( 'NONE',  ( 184.6718750003414016, 9.264065473108010111E-16, -7.564683531250000925 ) ) ;
#104815=CARTESIAN_POINT ( 'NONE',  ( 186.9427083336747160, -6.551208109652278289, 3.782341765624995134 ) ) ;
#104998=ADVANCED_FACE ( 'NONE', ( #55975 ), #116186, .T. ) ;
#105031=ORIENTED_EDGE ( 'NONE', *, *, #103912, .F. ) ;
#105040=CARTESIAN_POINT ( 'NONE',  ( 185.6093750003413732, 9.264065473108010111E-16, -7.564683531250000925 ) ) ;
#105098=CARTESIAN_POINT ( 'NONE',  ( 185.8593750003413732, 0.000000000000000000, 7.564683531250000925 ) ) ;
#105279=LINE ( 'NONE', #17526, #117752 ) ;
#105366=DIRECTION ( 'NONE',  ( 1.000000000000000000, 0.000000000000000000, 0.000000000000000000 ) ) ;
#105383=CARTESIAN_POINT ( 'NONE',  ( 187.5000000000000000, 0.000000000000000000, 0.000000000000000000 ) ) ;
#105424=EDGE_CURVE ( 'NONE', #87604, #109569, #25985, .T. ) ;
#105456=CARTESIAN_POINT ( 'NONE',  ( 185.0885416670080872, -6.551208109652273848, -3.782341765625003571 ) ) ;
#105458=CARTESIAN_POINT ( 'NONE',  ( 184.8385416670080872, 6.551208109652274736, 3.782341765625001351 ) ) ;
#105475=ORIENTED_EDGE ( 'NONE', *, *, #124411, .T. ) ;
#105547=FACE_OUTER_BOUND ( 'NONE', #84787, .T. ) ;
#105710=CARTESIAN_POINT ( 'NONE',  ( 187.2135416670080588, 4.367472073101518859, -7.564683531249999149 ) ) ;
#105750=LINE ( 'NONE', #16053, #126178 ) ;
#105763=CARTESIAN_POINT ( 'NONE',  ( 184.8593750003413732, 0.000000000000000000, 7.564683531250000925 ) ) ;
#105942=CYLINDRICAL_SURFACE ( 'NONE', #57382, 7.699999999999999289 ) ;
#105974=AXIS2_PLACEMENT_3D ( 'NONE', #13048, #62827, #60885 ) ;
#106096=CARTESIAN_POINT ( 'NONE',  ( 187.2916666666666572, 4.445597072760120838, -7.699999999999998401 ) ) ;
#106098=CARTESIAN_POINT ( 'NONE',  ( 185.0885416670080872, -6.551208109652273848, -3.782341765625003571 ) ) ;
#106128=CARTESIAN_POINT ( 'NONE',  ( 186.8593750003414016, 0.000000000000000000, 7.564683531250000925 ) ) ;
#106140=EDGE_LOOP ( 'NONE', ( #39540, #21524, #58108, #16967 ) ) ;
#106194=CARTESIAN_POINT ( 'NONE',  ( 185.2500000000000000, 9.429780353434619030E-16, -7.700000000000000178 ) ) ;
#106258=CARTESIAN_POINT ( 'NONE',  ( 185.1979166673494603, 6.668395609140176816, 3.850000000000000977 ) ) ;
#106344=CARTESIAN_POINT ( 'NONE',  ( 185.9218750003414016, 0.000000000000000000, 7.564683531250000925 ) ) ;
#106396=CARTESIAN_POINT ( 'NONE',  ( 185.5677083336747160, -4.367472073101514418, -7.564683531250002702 ) ) ;
#106469=EDGE_LOOP ( 'NONE', ( #44988, #19126, #109860, #1386, #42774 ) ) ;
#106620=VECTOR ( 'NONE', #88925, 1000.000000000000000 ) ;
#106626=PRODUCT_CONTEXT ( 'NONE', #53873, 'mechanical' ) ;
#106726=CARTESIAN_POINT ( 'NONE',  ( 187.2500000000000000, 9.429780353434619030E-16, -7.700000000000000178 ) ) ;
#106969=CARTESIAN_POINT ( 'NONE',  ( 183.8593750003413732, 0.000000000000000000, 7.564683531250000925 ) ) ;
#107039=CARTESIAN_POINT ( 'NONE',  ( 186.5312500006828031, 9.429780353434619030E-16, -7.700000000000000178 ) ) ;
#107184=ORIENTED_EDGE ( 'NONE', *, *, #64751, .T. ) ;
#107186=ORIENTED_EDGE ( 'NONE', *, *, #125920, .F. ) ;
#107200=DIRECTION ( 'NONE',  ( 1.000000000000000000, -0.000000000000000000, -0.000000000000000000 ) ) ;
#107227=LINE ( 'NONE', #98052, #53369 ) ;
#107347=CARTESIAN_POINT ( 'NONE',  ( 186.2395833340161175, 4.445597072760147483, 7.699999999999948663 ) ) ;
#107382=CARTESIAN_POINT ( 'NONE',  ( 185.9166666666666856, 6.668395609140176816, 3.850000000000000977 ) ) ;
#107432=SURFACE_STYLE_USAGE ( .BOTH. , #119188 ) ;
#107472=CARTESIAN_POINT ( 'NONE',  ( 186.1250000000000000, -8.891194145520236347, -1.633285867636356299E-15 ) ) ;
#107555=ORIENTED_EDGE ( 'NONE', *, *, #61987, .F. ) ;
#107593=CARTESIAN_POINT ( 'NONE',  ( 187.1979166673494603, 6.668395609140176816, 3.850000000000000977 ) ) ;
#107638=CARTESIAN_POINT ( 'NONE',  ( 185.6302083336747444, -4.367472073101514418, -7.564683531250002702 ) ) ;
#107833=FACE_OUTER_BOUND ( 'NONE', #112474, .T. ) ;
#107847=CARTESIAN_POINT ( 'NONE',  ( 187.2395833340161460, 4.445597072760117285, 7.699999999999999289 ) ) ;
#107890=CARTESIAN_POINT ( 'NONE',  ( 186.6979166673494603, 6.668395609140176816, 3.850000000000000977 ) ) ;
#107912=EDGE_LOOP ( 'NONE', ( #19522, #36621, #118276, #112246 ) ) ;
#107968=LINE ( 'NONE', #58866, #76258 ) ;
#108019=CARTESIAN_POINT ( 'NONE',  ( 184.2552083336747444, 6.551208109652275624, -3.782341765624998686 ) ) ;
#108189=VERTEX_POINT ( 'NONE', #99124 ) ;
#108228=CARTESIAN_POINT ( 'NONE',  ( 185.9583333333333144, 4.445597072760159030, 7.699999999999928235 ) ) ;
#108275=CARTESIAN_POINT ( 'NONE',  ( 186.3802083336747444, 4.367472073101515306, 7.564683531250000925 ) ) ;
#108290=PLANE ( 'NONE',  #16634 ) ;
#108296=AXIS2_PLACEMENT_3D ( 'NONE', #10644, #90516, #80718 ) ;
#108407=LINE ( 'NONE', #18741, #75476 ) ;
#108667=CARTESIAN_POINT ( 'NONE',  ( 185.5416666666666572, -4.445597072760122614, 7.699999999999998401 ) ) ;
#108701=CARTESIAN_POINT ( 'NONE',  ( 184.9010416670080588, -4.367472073101520635, 7.564683531249999149 ) ) ;
#108770=EDGE_LOOP ( 'NONE', ( #124523, #90663, #16681, #103904 ) ) ;
#108860=CARTESIAN_POINT ( 'NONE',  ( 185.7916666666666856, 4.445597072760072876, -7.700000000000080114 ) ) ;
#109023=CARTESIAN_POINT ( 'NONE',  ( 185.0312500006828031, 9.429780353434619030E-16, -7.700000000000000178 ) ) ;
#109166=CARTESIAN_POINT ( 'NONE',  ( 186.5729166673494888, 4.445597072760099522, -7.700000000000035705 ) ) ;
#109312=CARTESIAN_POINT ( 'NONE',  ( 184.2500000000000000, 9.429780353434619030E-16, -7.700000000000000178 ) ) ;
#109344=CARTESIAN_POINT ( 'NONE',  ( 184.5000000000000000, -7.430520870378829024, -1.418378131116527108 ) ) ;
#109381=CARTESIAN_POINT ( 'NONE',  ( 186.9895833340161744, -4.445597072760123503, -7.699999999999989519 ) ) ;
#109439=( BOUNDED_CURVE ( )  B_SPLINE_CURVE ( 2, ( #95645, #112717, #83260, #103543, #114628, #124466, #35447 ),
 .UNSPECIFIED., .F., .F. ) 
 B_SPLINE_CURVE_WITH_KNOTS ( ( 3, 2, 2, 3 ),
 ( 0.000000000000000000, 0.02380952380952383249, 0.04761904761904766498, 0.07142857142857149400 ),
 .UNSPECIFIED. ) 
 CURVE ( )  GEOMETRIC_REPRESENTATION_ITEM ( )  RATIONAL_B_SPLINE_CURVE ( ( 1.000000000000000000, 0.8660254037844387076, 1.000000000000000000, 0.8660254037844387076, 1.000000000000000000, 0.8660254037844383745, 1.000000000000000444 ) ) 
 REPRESENTATION_ITEM ( '' )  );
#109538=ORIENTED_EDGE ( 'NONE', *, *, #112824, .F. ) ;
#109544=ORIENTED_EDGE ( 'NONE', *, *, #66111, .F. ) ;
#109569=VERTEX_POINT ( 'NONE', #104291 ) ;
#109660=CARTESIAN_POINT ( 'NONE',  ( 184.4999999999999716, -0.6202644670797828885, 7.670962774272589435 ) ) ;
#109689=VERTEX_POINT ( 'NONE', #94452 ) ;
#109785=CARTESIAN_POINT ( 'NONE',  ( 186.8645833340161175, -6.668395609140180369, 3.849999999999994760 ) ) ;
#109860=ORIENTED_EDGE ( 'NONE', *, *, #72761, .T. ) ;
#109884=CARTESIAN_POINT ( 'NONE',  ( 195.5000000000000000, 0.000000000000000000, 0.000000000000000000 ) ) ;
#109898=ORIENTED_EDGE ( 'NONE', *, *, #62571, .F. ) ;
#109907=DIRECTION ( 'NONE',  ( 0.000000000000000000, 0.000000000000000000, 1.000000000000000000 ) ) ;
#109970=CARTESIAN_POINT ( 'NONE',  ( 185.0000000000000000, 0.000000000000000000, 7.700000000000000178 ) ) ;
#110038=CARTESIAN_POINT ( 'NONE',  ( 186.9062500006828316, -8.891194145520236347, -1.633285867636356299E-15 ) ) ;
#110172=EDGE_CURVE ( 'NONE', #1307, #70184, #41261, .T. ) ;
#110203=CARTESIAN_POINT ( 'NONE',  ( 185.0000000000000000, 0.000000000000000000, 7.700000000000000178 ) ) ;
#110271=DIRECTION ( 'NONE',  ( 0.000000000000000000, 0.000000000000000000, -1.000000000000000000 ) ) ;
#110273=( GEOMETRIC_REPRESENTATION_CONTEXT ( 3 ) GLOBAL_UNCERTAINTY_ASSIGNED_CONTEXT ( ( #113553 ) ) GLOBAL_UNIT_ASSIGNED_CONTEXT ( ( #87993, #67056, #17311 ) ) REPRESENTATION_CONTEXT ( 'NONE', 'WORKASPACE' ) );
#110420=CARTESIAN_POINT ( 'NONE',  ( 186.0312500006828031, 9.429780353434619030E-16, -7.700000000000000178 ) ) ;
#110601=CARTESIAN_POINT ( 'NONE',  ( 185.1666666666666856, -6.668395609140176816, -3.850000000000003642 ) ) ;
#110610=CYLINDRICAL_SURFACE ( 'NONE', #124139, 4.000000000000000000 ) ;
#110698=CARTESIAN_POINT ( 'NONE',  ( 195.0000000000000000, 0.000000000000000000, -3.500000000000000000 ) ) ;
#110926=CARTESIAN_POINT ( 'NONE',  ( 184.5000000000000000, -1.234829786877245983, 7.585434706901270197 ) ) ;
#110953=( BOUNDED_SURFACE ( )  B_SPLINE_SURFACE ( 1, 2, ( 
 ( #80665, #62317, #102235, #70831, #42691, #82600, #94324, #74056, #113986, #123779, #64866, #104782, #72769, #54409, #114615, #23028, #4639, #85797, #102853, #44599, #34141, #83864, #104160, #4014, #112699, #35432, #84520, #15099, #124449, #55062, #5938, #94993, #5301, #23667, #45247, #65517, #34798, #32867, #103522, #43961, #13832, #24311, #125088, #53768, #74702, #64233, #14466, #13181, #53134, #85162, #24954, #75334, #25582, #115230, #3378, #93065, #105456, #15766, #63601, #55697, #33505, #95633, #45892, #62943, #93696, #43325, #83245, #123161, #73401, #113328, #96909, #68093, #68745, #75986, #57647, #16393, #108019, #49131, #86442, #8518, #76638, #7884, #56338, #96254, #9183 ),
 ( #87729, #56974, #115907, #77278, #17023, #106096, #106726, #58934, #116551, #98842, #26893, #37996, #17699, #37372, #117172, #66796, #126384, #36726, #7227, #77913, #97557, #47185, #28185, #26254, #87085, #18355, #125710, #58299, #88365, #6564, #127664, #47836, #127041, #66159, #27511, #46515, #117827, #67422, #107382, #36068, #98201, #48463, #128336, #38670, #78592, #118481, #28837, #108667, #18987, #1928, #20939, #119139, #12396, #101433, #81156, #51697, #110601, #91609, #90969, #29473, #109970, #120430, #60861, #89038, #128987, #32066, #20294, #41883, #9826, #19654, #39323, #79226, #129617, #69382, #41241, #111225, #49777, #31413, #109312, #59605, #51060, #30778, #81774, #99514, #89679 ) ),
 .UNSPECIFIED., .F., .F., .F. ) 
 B_SPLINE_SURFACE_WITH_KNOTS ( ( 2, 2 ),
 ( 3, 2, 2, 2, 2, 2, 2, 2, 2, 2, 2, 2, 2, 2, 2, 2, 2, 2, 2, 2, 2, 2, 2, 2, 2, 2, 2, 2, 2, 2, 2, 2, 2, 2, 2, 2, 2, 2, 2, 2, 2, 2, 3 ),
 ( 0.000000000000000000, 1.000000000000000000 ),
 ( 0.000000000000000000, 0.02380952380952380820, 0.04761904761904761640, 0.07142857142857142461, 0.09523809523809523281, 0.1190476190476190410, 0.1428571428571428492, 0.1666666666666666574, 0.1904761904761904656, 0.2142857142857142738, 0.2380952380952380820, 0.2619047619047619180, 0.2857142857142856984, 0.3095238095238095344, 0.3333333333333333148, 0.3571428571428571508, 0.3809523809523809312, 0.4047619047619047672, 0.4285714285714285476, 0.4523809523809523836, 0.4761904761904761640, 0.5000000000000000000, 0.5238095238095238360, 0.5476190476190476719, 0.5714285714285713969, 0.5952380952380952328, 0.6190476190476190688, 0.6428571428571429047, 0.6666666666666666297, 0.6904761904761904656, 0.7142857142857143016, 0.7380952380952381375, 0.7619047619047618625, 0.7857142857142856984, 0.8095238095238095344, 0.8333333333333333703, 0.8571428571428570953, 0.8809523809523809312, 0.9047619047619047672, 0.9285714285714286031, 0.9523809523809523281, 0.9761904761904761640, 1.000000000000000000 ),
 .UNSPECIFIED. ) 
 GEOMETRIC_REPRESENTATION_ITEM ( )  RATIONAL_B_SPLINE_SURFACE ( (
 ( 1.000000000000000000, 0.8660254037844387076, 1.000000000000000000, 0.8660254037844387076, 1.000000000000000000, 0.8660254037844387076, 1.000000000000000000, 0.8660254037844387076, 1.000000000000000000, 0.8660254037844387076, 1.000000000000000000, 0.8660254037844387076, 1.000000000000000000, 0.8660254037844387076, 1.000000000000000000, 0.8660254037844387076, 1.000000000000000000, 0.8660254037844387076, 1.000000000000000000, 0.8660254037844387076, 1.000000000000000000, 0.8660254037844387076, 1.000000000000000000, 0.8660254037844387076, 1.000000000000000000, 0.8660254037844387076, 1.000000000000000000, 0.8660254037844387076, 1.000000000000000000, 0.8660254037844387076, 1.000000000000000000, 0.8660254037844387076, 1.000000000000000000, 0.8660254037844387076, 1.000000000000000000, 0.8660254037844387076, 1.000000000000000000, 0.8660254037844387076, 1.000000000000000000, 0.8660254037844387076, 1.000000000000000000, 0.8660254037844387076, 1.000000000000000000, 0.8660254037844387076, 1.000000000000000000, 0.8660254037844387076, 1.000000000000000000, 0.8660254037844387076, 1.000000000000000000, 0.8660254037844387076, 1.000000000000000000, 0.8660254037844387076, 1.000000000000000000, 0.8660254037844387076, 1.000000000000000000, 0.8660254037844387076, 1.000000000000000000, 0.8660254037844387076, 1.000000000000000000, 0.8660254037844387076, 1.000000000000000000, 0.8660254037844387076, 1.000000000000000000, 0.8660254037844387076, 1.000000000000000000, 0.8660254037844387076, 1.000000000000000000, 0.8660254037844387076, 1.000000000000000000, 0.8660254037844387076, 1.000000000000000000, 0.8660254037844387076, 1.000000000000000000, 0.8660254037844387076, 1.000000000000000000, 0.8660254037844387076, 1.000000000000000000, 0.8660254037844387076, 1.000000000000000000, 0.8660254037844387076, 1.000000000000000000, 0.8660254037844387076, 1.000000000000000000, 0.8660254037844387076, 1.000000000000000000),
 ( 1.000000000000000000, 0.8660254037844387076, 1.000000000000000000, 0.8660254037844387076, 1.000000000000000000, 0.8660254037844387076, 1.000000000000000000, 0.8660254037844387076, 1.000000000000000000, 0.8660254037844387076, 1.000000000000000000, 0.8660254037844387076, 1.000000000000000000, 0.8660254037844387076, 1.000000000000000000, 0.8660254037844387076, 1.000000000000000000, 0.8660254037844387076, 1.000000000000000000, 0.8660254037844387076, 1.000000000000000000, 0.8660254037844387076, 1.000000000000000000, 0.8660254037844387076, 1.000000000000000000, 0.8660254037844387076, 1.000000000000000000, 0.8660254037844387076, 1.000000000000000000, 0.8660254037844387076, 1.000000000000000000, 0.8660254037844387076, 1.000000000000000000, 0.8660254037844387076, 1.000000000000000000, 0.8660254037844387076, 1.000000000000000000, 0.8660254037844387076, 1.000000000000000000, 0.8660254037844387076, 1.000000000000000000, 0.8660254037844387076, 1.000000000000000000, 0.8660254037844387076, 1.000000000000000000, 0.8660254037844387076, 1.000000000000000000, 0.8660254037844387076, 1.000000000000000000, 0.8660254037844387076, 1.000000000000000000, 0.8660254037844387076, 1.000000000000000000, 0.8660254037844387076, 1.000000000000000000, 0.8660254037844387076, 1.000000000000000000, 0.8660254037844387076, 1.000000000000000000, 0.8660254037844387076, 1.000000000000000000, 0.8660254037844387076, 1.000000000000000000, 0.8660254037844387076, 1.000000000000000000, 0.8660254037844387076, 1.000000000000000000, 0.8660254037844387076, 1.000000000000000000, 0.8660254037844387076, 1.000000000000000000, 0.8660254037844387076, 1.000000000000000000, 0.8660254037844387076, 1.000000000000000000, 0.8660254037844387076, 1.000000000000000000, 0.8660254037844387076, 1.000000000000000000, 0.8660254037844387076, 1.000000000000000000, 0.8660254037844387076, 1.000000000000000000, 0.8660254037844387076, 1.000000000000000000) ) ) 
 REPRESENTATION_ITEM ( '' )  SURFACE ( )  );
#111002=ORIENTED_EDGE ( 'NONE', *, *, #56793, .T. ) ;
#111041=CARTESIAN_POINT ( 'NONE',  ( 187.1927083336747160, 6.551208109652275624, -3.782341765624998686 ) ) ;
#111063=DIRECTION ( 'NONE',  ( 0.000000000000000000, 0.000000000000000000, -1.000000000000000000 ) ) ;
#111079=CARTESIAN_POINT ( 'NONE',  ( 185.0312500006828031, 9.429780353434619030E-16, -7.700000000000000178 ) ) ;
#111111=CARTESIAN_POINT ( 'NONE',  ( 184.7812500006828031, 0.000000000000000000, 7.700000000000000178 ) ) ;
#111171=AXIS2_PLACEMENT_3D ( 'NONE', #43798, #4463, #55539 ) ;
#111174=AXIS2_PLACEMENT_3D ( 'NONE', #22652, #63204, #12791 ) ;
#111225=CARTESIAN_POINT ( 'NONE',  ( 184.3750000000000000, 8.891194145520236347, 5.444286225454521982E-16 ) ) ;
#111285=ADVANCED_FACE ( 'NONE', ( #100291, #1430 ), #91752, .T. ) ;
#111312=CARTESIAN_POINT ( 'NONE',  ( 185.2812500006828031, 0.000000000000000000, 7.700000000000000178 ) ) ;
#111582=DIRECTION ( 'NONE',  ( -1.000000000000000000, 0.000000000000000000, 0.000000000000000000 ) ) ;
#111669=CYLINDRICAL_SURFACE ( 'NONE', #111174, 7.699999999999999289 ) ;
#111715=CARTESIAN_POINT ( 'NONE',  ( 184.6979166673494603, 6.668395609140176816, 3.850000000000000977 ) ) ;
#111842=CARTESIAN_POINT ( 'NONE',  ( 184.5166856079987667, -1.553938115584203139, -7.699999999999964650 ) ) ;
#112015=CARTESIAN_POINT ( 'NONE',  ( 184.4999999999999716, -6.820224004183075728, 3.418167119943706034 ) ) ;
#112111=CARTESIAN_POINT ( 'NONE',  ( 185.3229166673494888, -4.445597072760063107, 7.700000000000102318 ) ) ;
#112144=CARTESIAN_POINT ( 'NONE',  ( 183.9843750003414016, -8.734944146203032389, -1.604583208406768146E-15 ) ) ;
#112246=ORIENTED_EDGE ( 'NONE', *, *, #34914, .F. ) ;
#112290=ORIENTED_EDGE ( 'NONE', *, *, #124411, .F. ) ;
#112306=CARTESIAN_POINT ( 'NONE',  ( 186.3593750003414016, 0.000000000000000000, 7.564683531250000925 ) ) ;
#112364=ORIENTED_EDGE ( 'NONE', *, *, #59537, .F. ) ;
#112366=CARTESIAN_POINT ( 'NONE',  ( 184.1562500006828316, 8.891194145520236347, 5.444286225454521982E-16 ) ) ;
#112440=EDGE_LOOP ( 'NONE', ( #19263, #22943 ) ) ;
#112474=EDGE_LOOP ( 'NONE', ( #78308, #100432, #22767 ) ) ;
#112552=DIRECTION ( 'NONE',  ( 1.000000000000000000, -0.000000000000000000, -0.000000000000000000 ) ) ;
#112666=CARTESIAN_POINT ( 'NONE',  ( 187.2083333333333712, -4.445597072760123503, -7.699999999999989519 ) ) ;
#112699=CARTESIAN_POINT ( 'NONE',  ( 186.4218750003414016, 0.000000000000000000, 7.564683531250000925 ) ) ;
#112717=CARTESIAN_POINT ( 'NONE',  ( 187.4583333333333428, 4.445597072760117285, 7.700000000000001066 ) ) ;
#112790=CARTESIAN_POINT ( 'NONE',  ( 183.9427083336747160, -6.551208109652278289, 3.782341765624995134 ) ) ;
#112824=EDGE_CURVE ( 'NONE', #67674, #100903, #5109, .T. ) ;
#112882=CARTESIAN_POINT ( 'NONE',  ( 185.3333333333333144, 6.668395609140177704, -3.849999999999998312 ) ) ;
#112944=CARTESIAN_POINT ( 'NONE',  ( 186.0677083336747444, -4.367472073101514418, -7.564683531250002702 ) ) ;
#113000=CARTESIAN_POINT ( 'NONE',  ( 183.9062500006828031, -8.891194145520236347, -1.633285867636356693E-15 ) ) ;
#113050=DIRECTION ( 'NONE',  ( 0.000000000000000000, 0.000000000000000000, -1.000000000000000000 ) ) ;
#113189=DIRECTION ( 'NONE',  ( 1.000000000000000000, -0.000000000000000000, -0.000000000000000000 ) ) ;
#113195=EDGE_LOOP ( 'NONE', ( #87166, #53261, #14025, #111002 ) ) ;
#113328=CARTESIAN_POINT ( 'NONE',  ( 184.5468750003414300, -8.734944146203032389, -1.604583208406768146E-15 ) ) ;
#113335=AXIS2_PLACEMENT_3D ( 'NONE', #128411, #66230, #48538 ) ;
#113364=CARTESIAN_POINT ( 'NONE',  ( 186.1510416670080588, 4.367472073101518859, -7.564683531249999149 ) ) ;
#113380=CARTESIAN_POINT ( 'NONE',  ( 186.9166666666666856, 6.668395609140176816, 3.850000000000000977 ) ) ;
#113553=UNCERTAINTY_MEASURE_WITH_UNIT (LENGTH_MEASURE( 1.000000000000000082E-05 ), #87993, 'distance_accuracy_value', 'NONE');
#113592=CARTESIAN_POINT ( 'NONE',  ( 184.9010416670080588, -4.367472073101519747, 7.564683531249999149 ) ) ;
#113643=( BOUNDED_CURVE ( )  B_SPLINE_CURVE ( 2, ( #122949, #111842, #14263 ),
 .UNSPECIFIED., .F., .F. ) 
 B_SPLINE_CURVE_WITH_KNOTS ( ( 3, 3 ),
 ( 0.7857142857142862535, 0.7948312917401810784 ),
 .UNSPECIFIED. ) 
 CURVE ( )  GEOMETRIC_REPRESENTATION_ITEM ( )  RATIONAL_B_SPLINE_CURVE ( ( 0.9999999999999968914, 0.9486992175574040509, 0.9366860366984419706 ) ) 
 REPRESENTATION_ITEM ( '' )  );
#113644=CARTESIAN_POINT ( 'NONE',  ( 186.2500000000000000, 9.429780353434619030E-16, -7.700000000000000178 ) ) ;
#113647=CARTESIAN_POINT ( 'NONE',  ( 184.7812500006828031, 0.000000000000000000, 7.700000000000000178 ) ) ;
#113703=DIRECTION ( 'NONE',  ( 0.000000000000000000, 0.000000000000000000, -1.000000000000000000 ) ) ;
#113712=CARTESIAN_POINT ( 'NONE',  ( 184.4999999999999716, -5.087293621995115700, -5.751705878905746694 ) ) ;
#113763=ORIENTED_EDGE ( 'NONE', *, *, #26068, .F. ) ;
#113907=CARTESIAN_POINT ( 'NONE',  ( 186.5416666666666572, -4.445597072760092416, 7.700000000000049916 ) ) ;
#113944=ADVANCED_FACE ( 'NONE', ( #33337 ), #124919, .F. ) ;
#113986=CARTESIAN_POINT ( 'NONE',  ( 187.0885416670080872, -6.551208109652273848, -3.782341765625003571 ) ) ;
#113988=CARTESIAN_POINT ( 'NONE',  ( 184.7135416670080588, 4.367472073101518859, -7.564683531249999149 ) ) ;
#114022=CARTESIAN_POINT ( 'NONE',  ( 187.1927083336747160, 6.551208109652275624, -3.782341765624998686 ) ) ;
#114067=CARTESIAN_POINT ( 'NONE',  ( 186.0312500006828031, 9.429780353434619030E-16, -7.700000000000000178 ) ) ;
#114072=CARTESIAN_POINT ( 'NONE',  ( 184.2760416670080588, 6.551208109652274736, 3.782341765625001351 ) ) ;
#114235=CARTESIAN_POINT ( 'NONE',  ( 186.6510416670080303, 4.367472073101518859, -7.564683531249999149 ) ) ;
#114283=CARTESIAN_POINT ( 'NONE',  ( 186.2343750003414016, 8.734944146203032389, 5.348610694689227483E-16 ) ) ;
#114415=DIRECTION ( 'NONE',  ( 0.000000000000000000, 0.000000000000000000, -1.000000000000000000 ) ) ;
#114471=VECTOR ( 'NONE', #84134, 1000.000000000000000 ) ;
#114511=DIRECTION ( 'NONE',  ( 0.000000000000000000, 0.000000000000000000, -1.000000000000000000 ) ) ;
#114615=CARTESIAN_POINT ( 'NONE',  ( 186.8385416670080872, 6.551208109652274736, 3.782341765625001351 ) ) ;
#114617=CARTESIAN_POINT ( 'NONE',  ( 185.8385416670080872, 6.551208109652274736, 3.782341765625001351 ) ) ;
#114628=CARTESIAN_POINT ( 'NONE',  ( 187.3333333333333144, 6.668395609140177704, -3.849999999999998312 ) ) ;
#114863=CARTESIAN_POINT ( 'NONE',  ( 186.8593750003414016, 0.000000000000000000, 7.564683531250000925 ) ) ;
#114868=EDGE_CURVE ( 'NONE', #36662, #91613, #102701, .T. ) ;
#114918=CARTESIAN_POINT ( 'NONE',  ( 185.0260416670080588, -6.551208109652273848, -3.782341765625003571 ) ) ;
#115078=AXIS2_PLACEMENT_3D ( 'NONE', #19973, #59270, #58615 ) ;
#115134=LINE ( 'NONE', #65413, #10977 ) ;
#115224=AXIS2_PLACEMENT_3D ( 'NONE', #109884, #87643, #37909 ) ;
#115230=CARTESIAN_POINT ( 'NONE',  ( 185.2135416670080872, 4.367472073101518859, -7.564683531249999149 ) ) ;
#115233=CARTESIAN_POINT ( 'NONE',  ( 184.9218750003414016, 0.000000000000000000, 7.564683531250000925 ) ) ;
#115267=CARTESIAN_POINT ( 'NONE',  ( 186.7760416670080588, 6.551208109652274736, 3.782341765625001351 ) ) ;
#115397=CARTESIAN_POINT ( 'NONE',  ( 185.2812500006828031, 0.000000000000000000, 7.700000000000000178 ) ) ;
#115425=ADVANCED_FACE ( 'NONE', ( #80126 ), #61129, .T. ) ;
#115498=CARTESIAN_POINT ( 'NONE',  ( 184.1093750003413732, 9.264065473108010111E-16, -7.564683531250000925 ) ) ;
#115554=CARTESIAN_POINT ( 'NONE',  ( 185.0677083336747160, -4.367472073101514418, -7.564683531250002702 ) ) ;
#115907=CARTESIAN_POINT ( 'NONE',  ( 187.4166666666666856, 6.668395609140176816, 3.850000000000000977 ) ) ;
#115928=ORIENTED_EDGE ( 'NONE', *, *, #17985, .T. ) ;
#116114=CARTESIAN_POINT ( 'NONE',  ( 184.5000000000000000, 9.429780353434619030E-16, 7.699999999999999289 ) ) ;
#116131=CARTESIAN_POINT ( 'NONE',  ( 187.3906250003414016, 0.000000000000000000, 7.564683531250000925 ) ) ;
#116152=CARTESIAN_POINT ( 'NONE',  ( 187.1718750003414016, 9.264065473108010111E-16, -7.564683531250000925 ) ) ;
#116186=CYLINDRICAL_SURFACE ( 'NONE', #63543, 7.699999999999999289 ) ;
#116209=CARTESIAN_POINT ( 'NONE',  ( 185.7343750003414016, 8.734944146203032389, 5.348610694689227483E-16 ) ) ;
#116520=CARTESIAN_POINT ( 'NONE',  ( 186.0312500006828031, 9.429780353434619030E-16, -7.700000000000000178 ) ) ;
#116551=CARTESIAN_POINT ( 'NONE',  ( 187.1666666666666856, -6.668395609140176816, -3.850000000000003642 ) ) ;
#116753=CARTESIAN_POINT ( 'NONE',  ( 187.1145833340161175, 6.668395609140177704, -3.849999999999998312 ) ) ;
#116794=CARTESIAN_POINT ( 'NONE',  ( 185.4218750003414016, 0.000000000000000000, 7.564683531250000925 ) ) ;
#116853=FACE_BOUND ( 'NONE', #99787, .T. ) ;
#117052=DIRECTION ( 'NONE',  ( 0.000000000000000000, 0.000000000000000000, -1.000000000000000000 ) ) ;
#117172=CARTESIAN_POINT ( 'NONE',  ( 186.9166666666666856, 6.668395609140176816, 3.850000000000000977 ) ) ;
#117178=VERTEX_POINT ( 'NONE', #31814 ) ;
#117419=CARTESIAN_POINT ( 'NONE',  ( 186.2968750003414584, 8.734944146203032389, 5.348610694689227483E-16 ) ) ;
#117440=SURFACE_STYLE_FILL_AREA ( #19258 ) ;
#117591=DIRECTION ( 'NONE',  ( 0.000000000000000000, 0.000000000000000000, 1.000000000000000000 ) ) ;
#117639=CARTESIAN_POINT ( 'NONE',  ( 186.8229166673494319, -4.445597072760122614, 7.699999999999998401 ) ) ;
#117714=CARTESIAN_POINT ( 'NONE',  ( 187.2812500006828031, 0.000000000000000000, 7.700000000000000178 ) ) ;
#117726=CARTESIAN_POINT ( 'NONE',  ( 184.5312500006828031, 9.429780353434619030E-16, -7.700000000000000178 ) ) ;
#117737=DIRECTION ( 'NONE',  ( 0.000000000000000000, 0.000000000000000000, -1.000000000000000000 ) ) ;
#117752=VECTOR ( 'NONE', #107200, 1000.000000000000000 ) ;
#117805=LINE ( 'NONE', #129608, #51062 ) ;
#117824=( BOUNDED_CURVE ( )  B_SPLINE_CURVE ( 2, ( #123835, #13235, #102289, #23080, #14524, #112111, #63001 ),
 .UNSPECIFIED., .F., .F. ) 
 B_SPLINE_CURVE_WITH_KNOTS ( ( 3, 2, 2, 3 ),
 ( 0.5000000000000004441, 0.5238095238095242800, 0.5476190476190482270, 0.5714285714285719520 ),
 .UNSPECIFIED. ) 
 CURVE ( )  GEOMETRIC_REPRESENTATION_ITEM ( )  RATIONAL_B_SPLINE_CURVE ( ( 0.9999999999999974465, 0.8660254037844412611, 1.000000000000000000, 0.8660254037844387076, 1.000000000000000000, 0.8660254037844355990, 1.000000000000003109 ) ) 
 REPRESENTATION_ITEM ( '' )  );
#117827=CARTESIAN_POINT ( 'NONE',  ( 186.0000000000000000, 0.000000000000000000, 7.700000000000000178 ) ) ;
#117864=CARTESIAN_POINT ( 'NONE',  ( 185.3177083336747160, 4.367472073101515306, 7.564683531250000925 ) ) ;
#118090=CARTESIAN_POINT ( 'NONE',  ( 186.8802083336747444, 4.367472073101515306, 7.564683531250000925 ) ) ;
#118172=ORIENTED_EDGE ( 'NONE', *, *, #124808, .F. ) ;
#118276=ORIENTED_EDGE ( 'NONE', *, *, #124808, .T. ) ;
#118353=CARTESIAN_POINT ( 'NONE',  ( 186.7395833340161175, 4.445597072760133273, 7.699999999999975309 ) ) ;
#118481=CARTESIAN_POINT ( 'NONE',  ( 185.6250000000000284, -8.891194145520236347, -1.633285867636356693E-15 ) ) ;
#118677=EDGE_LOOP ( 'NONE', ( #97035, #112290 ) ) ;
#118953=CARTESIAN_POINT ( 'NONE',  ( 186.1145833340161175, 6.668395609140177704, -3.849999999999998312 ) ) ;
#119003=CARTESIAN_POINT ( 'NONE',  ( 186.7812500006828031, 0.000000000000000000, 7.700000000000000178 ) ) ;
#119013=ADVANCED_FACE ( 'NONE', ( #101709 ), #58016, .T. ) ;
#119039=CARTESIAN_POINT ( 'NONE',  ( 195.0435778713738557, -1.025030745786872263E-15, 8.040022453829767102 ) ) ;
#119139=CARTESIAN_POINT ( 'NONE',  ( 185.3750000000000284, 8.891194145520236347, 5.444286225454521982E-16 ) ) ;
#119188=SURFACE_SIDE_STYLE ('',( #77967 ) ) ;
#119371=EDGE_LOOP ( 'NONE', ( #22459, #90508, #105475, #109538 ) ) ;
#119374=CARTESIAN_POINT ( 'NONE',  ( 184.0052083336747160, -6.551208109652278289, 3.782341765624995134 ) ) ;
#119528=CARTESIAN_POINT ( 'NONE',  ( 187.0260416670080588, -6.551208109652273848, -3.782341765625003571 ) ) ;
#119681=DIRECTION ( 'NONE',  ( 0.000000000000000000, 0.000000000000000000, 1.000000000000000000 ) ) ;
#119801=AXIS2_PLACEMENT_3D ( 'NONE', #45988, #125803, #36167 ) ;
#119847=CARTESIAN_POINT ( 'NONE',  ( 186.8645833340161175, -6.668395609140180369, 3.849999999999994760 ) ) ;
#120067=AXIS2_PLACEMENT_3D ( 'NONE', #78050, #125850, #97050 ) ;
#120185=ORIENTED_EDGE ( 'NONE', *, *, #87978, .T. ) ;
#120233=CARTESIAN_POINT ( 'NONE',  ( 184.7500000000000000, 9.429780353434619030E-16, -7.700000000000000178 ) ) ;
#120256=CARTESIAN_POINT ( 'NONE',  ( 186.3229166673494603, -4.445597072760122614, 7.699999999999998401 ) ) ;
#120294=CARTESIAN_POINT ( 'NONE',  ( 184.5000000000000000, -6.267304879582558996, 4.236192450104883100 ) ) ;
#120421=DIRECTION ( 'NONE',  ( 0.000000000000000000, 0.000000000000000000, -1.000000000000000000 ) ) ;
#120430=CARTESIAN_POINT ( 'NONE',  ( 184.9583333333333144, 4.445597072760117285, 7.699999999999999289 ) ) ;
#120682=CARTESIAN_POINT ( 'NONE',  ( 184.5885416670080872, -6.551208109652273848, -3.782341765625003571 ) ) ;
#120770=VERTEX_POINT ( 'NONE', #111111 ) ;
#120867=CARTESIAN_POINT ( 'NONE',  ( 184.5000000000000000, 0.000000000000000000, 7.700000000000000178 ) ) ;
#120883=CARTESIAN_POINT ( 'NONE',  ( 185.2395833340161175, 4.445597072760117285, 7.699999999999999289 ) ) ;
#121223=CARTESIAN_POINT ( 'NONE',  ( 187.2135416670080303, 4.367472073101518859, -7.564683531249999149 ) ) ;
#121317=CARTESIAN_POINT ( 'NONE',  ( 184.0885416670080872, -6.551208109652273848, -3.782341765625003571 ) ) ;
#121353=EDGE_CURVE ( 'NONE', #64176, #52063, #23906, .T. ) ;
#121458=CARTESIAN_POINT ( 'NONE',  ( 187.2343750003414016, 8.734944146203032389, 5.348610694689227483E-16 ) ) ;
#121512=CARTESIAN_POINT ( 'NONE',  ( 184.9062500006828031, -8.891194145520236347, -1.633285867636356693E-15 ) ) ;
#121542=CARTESIAN_POINT ( 'NONE',  ( 195.5000000000000000, 0.000000000000000000, 0.000000000000000000 ) ) ;
#121551=EDGE_LOOP ( 'NONE', ( #14851, #74677, #64928, #107184 ) ) ;
#121663=VERTEX_POINT ( 'NONE', #103433 ) ;
#121824=ORIENTED_EDGE ( 'NONE', *, *, #95250, .T. ) ;
#122132=CARTESIAN_POINT ( 'NONE',  ( 186.4843750003414016, -8.734944146203032389, -1.604583208406768146E-15 ) ) ;
#122188=CARTESIAN_POINT ( 'NONE',  ( 184.2395833340161175, 4.445597072760117285, 7.699999999999999289 ) ) ;
#122519=CARTESIAN_POINT ( 'NONE',  ( 187.0468750003414300, -8.734944146203032389, -1.604583208406767949E-15 ) ) ;
#122527=DIRECTION ( 'NONE',  ( -1.000000000000000000, 0.000000000000000000, 0.000000000000000000 ) ) ;
#122764=DIRECTION ( 'NONE',  ( 0.000000000000000000, 0.000000000000000000, -1.000000000000000000 ) ) ;
#122765=CARTESIAN_POINT ( 'NONE',  ( 186.8177083336747160, 4.367472073101515306, 7.564683531250000925 ) ) ;
#122827=CARTESIAN_POINT ( 'NONE',  ( 185.5312500006828031, 9.429780353434619030E-16, -7.700000000000000178 ) ) ;
#122867=LINE ( 'NONE', #72483, #16302 ) ;
#122878=ORIENTED_EDGE ( 'NONE', *, *, #30995, .T. ) ;
#122949=CARTESIAN_POINT ( 'NONE',  ( 184.5312500006828031, 9.429780353434619030E-16, -7.700000000000000178 ) ) ;
#123093=DIRECTION ( 'NONE',  ( 1.000000000000000000, 0.000000000000000000, 0.000000000000000000 ) ) ;
#123161=CARTESIAN_POINT ( 'NONE',  ( 184.6302083336747444, -4.367472073101514418, -7.564683531250002702 ) ) ;
#123165=CARTESIAN_POINT ( 'NONE',  ( 187.0052083336747444, -6.551208109652278289, 3.782341765624995134 ) ) ;
#123196=AXIS2_PLACEMENT_3D ( 'NONE', #29917, #40390, #80311 ) ;
#123246=CARTESIAN_POINT ( 'NONE',  ( 184.7916666666666572, 4.445597072760062218, -7.700000000000102318 ) ) ;
#123346=LINE ( 'NONE', #14015, #33033 ) ;
#123397=CARTESIAN_POINT ( 'NONE',  ( 185.6510416670080303, 4.367472073101518859, -7.564683531249999149 ) ) ;
#123453=CARTESIAN_POINT ( 'NONE',  ( 187.3593750003414016, 0.000000000000000000, 7.564683531250000925 ) ) ;
#123485=DIRECTION ( 'NONE',  ( 1.000000000000000000, -0.000000000000000000, -0.000000000000000000 ) ) ;
#123588=CARTESIAN_POINT ( 'NONE',  ( 184.5000000000000000, 0.000000000000000000, 0.000000000000000000 ) ) ;
#123627=ADVANCED_FACE ( 'NONE', ( #30985 ), #18556, .T. ) ;
#123779=CARTESIAN_POINT ( 'NONE',  ( 187.0468750003414300, -8.734944146203032389, -1.604583208406768146E-15 ) ) ;
#123781=CARTESIAN_POINT ( 'NONE',  ( 184.6302083336747444, -4.367472073101514418, -7.564683531250002702 ) ) ;
#123815=CARTESIAN_POINT ( 'NONE',  ( 184.5000000000000000, 0.000000000000000000, -7.699999999999999289 ) ) ;
#123817=CARTESIAN_POINT ( 'NONE',  ( 186.1093750003413732, 9.264065473108010111E-16, -7.564683531250000925 ) ) ;
#123834=CARTESIAN_POINT ( 'NONE',  ( 186.7500000000000000, 9.429780353434619030E-16, -7.700000000000000178 ) ) ;
#123835=CARTESIAN_POINT ( 'NONE',  ( 185.5312500006828031, 9.429780353434619030E-16, -7.700000000000000178 ) ) ;
#123873=CARTESIAN_POINT ( 'NONE',  ( 184.5677083336747444, -4.367472073101514418, -7.564683531250002702 ) ) ;
#123935=ORIENTED_EDGE ( 'NONE', *, *, #47594, .F. ) ;
#123972=CARTESIAN_POINT ( 'NONE',  ( 185.2500000000000000, 9.429780353434619030E-16, -7.700000000000000178 ) ) ;
#124030=LINE ( 'NONE', #55300, #68222 ) ;
#124046=CARTESIAN_POINT ( 'NONE',  ( 185.3177083336747160, 4.367472073101515306, 7.564683531250000925 ) ) ;
#124096=ORIENTED_EDGE ( 'NONE', *, *, #129551, .T. ) ;
#124103=CARTESIAN_POINT ( 'NONE',  ( 186.6510416670080303, 4.367472073101518859, -7.564683531249999149 ) ) ;
#124139=AXIS2_PLACEMENT_3D ( 'NONE', #28843, #60250, #18360 ) ;
#124159=DIRECTION ( 'NONE',  ( 1.000000000000000000, 0.000000000000000000, 0.000000000000000000 ) ) ;
#124256=ORIENTED_EDGE ( 'NONE', *, *, #94769, .F. ) ;
#124367=FACE_OUTER_BOUND ( 'NONE', #98472, .T. ) ;
#124411=EDGE_CURVE ( 'NONE', #65296, #100903, #66962, .T. ) ;
#124449=CARTESIAN_POINT ( 'NONE',  ( 186.2552083336747444, 6.551208109652275624, -3.782341765624998686 ) ) ;
#124462=VECTOR ( 'NONE', #127243, 1000.000000000000000 ) ;
#124466=CARTESIAN_POINT ( 'NONE',  ( 187.2916666666666572, 4.445597072760113733, -7.700000000000009948 ) ) ;
#124523=ORIENTED_EDGE ( 'NONE', *, *, #105424, .F. ) ;
#124664=ORIENTED_EDGE ( 'NONE', *, *, #28810, .T. ) ;
#124704=CARTESIAN_POINT ( 'NONE',  ( 184.3593750003413732, 0.000000000000000000, 7.564683531250000925 ) ) ;
#124755=CARTESIAN_POINT ( 'NONE',  ( 185.2343750003414016, 8.734944146203032389, 5.348610694689227483E-16 ) ) ;
#124808=EDGE_CURVE ( 'NONE', #54095, #8279, #41030, .T. ) ;
#124824=CARTESIAN_POINT ( 'NONE',  ( 184.4999999999999432, -5.532705916124244894, -5.308109601923121090 ) ) ;
#124919=PLANE ( 'NONE',  #111171 ) ;
#124939=DIRECTION ( 'NONE',  ( 0.000000000000000000, 0.000000000000000000, -1.000000000000000000 ) ) ;
#125041=CIRCLE ( 'NONE', #16352, 7.541925104783893552 ) ;
#125058=EDGE_CURVE ( 'NONE', #26135, #101886, #2389, .T. ) ;
#125088=CARTESIAN_POINT ( 'NONE',  ( 185.6718750003414016, 9.264065473108010111E-16, -7.564683531250000925 ) ) ;
#125090=CARTESIAN_POINT ( 'NONE',  ( 185.6302083336747444, -4.367472073101514418, -7.564683531250002702 ) ) ;
#125176=CARTESIAN_POINT ( 'NONE',  ( 185.8645833340161175, -6.668395609140180369, 3.849999999999994760 ) ) ;
#125231=CARTESIAN_POINT ( 'NONE',  ( 185.6145833340161175, 6.668395609140177704, -3.849999999999998312 ) ) ;
#125343=CARTESIAN_POINT ( 'NONE',  ( 186.2552083336747444, 6.551208109652275624, -3.782341765624998686 ) ) ;
#125401=CARTESIAN_POINT ( 'NONE',  ( 185.7760416670080588, 6.551208109652274736, 3.782341765625001351 ) ) ;
#125481=DIRECTION ( 'NONE',  ( 1.000000000000000000, -0.000000000000000000, -0.000000000000000000 ) ) ;
#125505=CARTESIAN_POINT ( 'NONE',  ( 187.5000000000000000, 0.000000000000000000, -8.699999999999999289 ) ) ;
#125547=CARTESIAN_POINT ( 'NONE',  ( 187.5000000000000000, 0.000000000000000000, 0.000000000000000000 ) ) ;
#125585=DIRECTION ( 'NONE',  ( 0.000000000000000000, 0.000000000000000000, -1.000000000000000000 ) ) ;
#125710=CARTESIAN_POINT ( 'NONE',  ( 186.4166666666666856, 6.668395609140176816, 3.850000000000000977 ) ) ;
#125713=CARTESIAN_POINT ( 'NONE',  ( 185.5468750003414300, -8.734944146203032389, -1.604583208406767949E-15 ) ) ;
#125803=DIRECTION ( 'NONE',  ( 1.000000000000000000, -0.000000000000000000, -0.000000000000000000 ) ) ;
#125805=AXIS2_PLACEMENT_3D ( 'NONE', #11938, #82634, #72808 ) ;
#125845=DIRECTION ( 'NONE',  ( 0.000000000000000000, 0.000000000000000000, -1.000000000000000000 ) ) ;
#125850=DIRECTION ( 'NONE',  ( 0.000000000000000000, 1.000000000000000000, -1.224646799147353207E-16 ) ) ;
#125920=EDGE_CURVE ( 'NONE', #52063, #108189, #101936, .T. ) ;
#125971=CARTESIAN_POINT ( 'NONE',  ( 186.3385416670080872, 6.551208109652274736, 3.782341765625001351 ) ) ;
#126027=CARTESIAN_POINT ( 'NONE',  ( 186.8593750003414016, 0.000000000000000000, 7.564683531250000925 ) ) ;
#126128=ORIENTED_EDGE ( 'NONE', *, *, #38452, .F. ) ;
#126178=VECTOR ( 'NONE', #6868, 1000.000000000000114 ) ;
#126299=CARTESIAN_POINT ( 'NONE',  ( 185.2083333333333144, -4.445597072760163471, -7.699999999999919353 ) ) ;
#126309=CARTESIAN_POINT ( 'NONE',  ( 186.7500000000000000, 9.429780353434619030E-16, -7.700000000000000178 ) ) ;
#126384=CARTESIAN_POINT ( 'NONE',  ( 186.8333333333333144, 6.668395609140177704, -3.849999999999998312 ) ) ;
#126417=CARTESIAN_POINT ( 'NONE',  ( 186.1927083336747160, 6.551208109652275624, -3.782341765624998686 ) ) ;
#126452=EDGE_LOOP ( 'NONE', ( #42521, #58129 ) ) ;
#126638=CARTESIAN_POINT ( 'NONE',  ( 186.8385416670080872, 6.551208109652274736, 3.782341765625001351 ) ) ;
#126863=EDGE_CURVE ( 'NONE', #79758, #32478, #16906, .T. ) ;
#127038=( BOUNDED_CURVE ( )  B_SPLINE_CURVE ( 2, ( #45392, #54534, #94464, #4788, #125231, #44748, #84661 ),
 .UNSPECIFIED., .F., .F. ) 
 B_SPLINE_CURVE_WITH_KNOTS ( ( 3, 2, 2, 3 ),
 ( 0.4285714285714289362, 0.4523809523809527722, 0.4761904761904766081, 0.5000000000000004441 ),
 .UNSPECIFIED. ) 
 CURVE ( )  GEOMETRIC_REPRESENTATION_ITEM ( )  RATIONAL_B_SPLINE_CURVE ( ( 0.9999999999999977796, 0.8660254037844409281, 1.000000000000000000, 0.8660254037844387076, 1.000000000000000000, 0.8660254037844361541, 1.000000000000002442 ) ) 
 REPRESENTATION_ITEM ( '' )  );
#127041=CARTESIAN_POINT ( 'NONE',  ( 186.1666666666666856, -6.668395609140176816, -3.850000000000003642 ) ) ;
#127068=CARTESIAN_POINT ( 'NONE',  ( 184.9843750003414016, -8.734944146203032389, -1.604583208406767949E-15 ) ) ;
#127169=ADVANCED_FACE ( 'NONE', ( #89552 ), #79106, .T. ) ;
#127243=DIRECTION ( 'NONE',  ( 1.000000000000000000, -0.000000000000000000, -0.000000000000000000 ) ) ;
#127244=CARTESIAN_POINT ( 'NONE',  ( 187.0312500006828031, 9.429780353434619030E-16, -7.700000000000000178 ) ) ;
#127287=CARTESIAN_POINT ( 'NONE',  ( 185.9635416670080872, -4.367472073101519747, 7.564683531249999149 ) ) ;
#127308=FILL_AREA_STYLE_COLOUR ( '', #58060 ) ;
#127368=CARTESIAN_POINT ( 'NONE',  ( 184.5000000000000000, -5.524290953051901099, 5.236943753751942765 ) ) ;
#127571=CARTESIAN_POINT ( 'NONE',  ( 184.6145833340161175, 6.668395609140177704, -3.849999999999998312 ) ) ;
#127664=CARTESIAN_POINT ( 'NONE',  ( 186.2500000000000000, 9.429780353434619030E-16, -7.700000000000000178 ) ) ;
#127918=CARTESIAN_POINT ( 'NONE',  ( 184.2343750003414016, 8.734944146203032389, 5.348610694689227483E-16 ) ) ;
#127995=EDGE_CURVE ( 'NONE', #52320, #108189, #19783, .T. ) ;
#128082=AXIS2_PLACEMENT_3D ( 'NONE', #86336, #47088, #114511 ) ;
#128311=CARTESIAN_POINT ( 'NONE',  ( 186.4062500006828031, -8.891194145520236347, -1.633285867636356299E-15 ) ) ;
#128336=CARTESIAN_POINT ( 'NONE',  ( 185.7500000000000000, 9.429780353434619030E-16, -7.700000000000000178 ) ) ;
#128353=CARTESIAN_POINT ( 'NONE',  ( 195.0000000000000000, 0.000000000000000000, -7.541925104783893552 ) ) ;
#128411=CARTESIAN_POINT ( 'NONE',  ( 194.5000000000000000, 0.000000000000000000, 0.000000000000000000 ) ) ;
#128418=ORIENTED_EDGE ( 'NONE', *, *, #102895, .T. ) ;
#128467=CARTESIAN_POINT ( 'NONE',  ( 184.5000000000000000, 6.368163355566236381E-16, 5.200000000000000178 ) ) ;
#128574=ORIENTED_EDGE ( 'NONE', *, *, #35369, .T. ) ;
#128593=CARTESIAN_POINT ( 'NONE',  ( 184.4218750003414016, 0.000000000000000000, 7.564683531250000925 ) ) ;
#128967=CARTESIAN_POINT ( 'NONE',  ( 186.2812500006828031, 0.000000000000000000, 7.700000000000000178 ) ) ;
#128987=CARTESIAN_POINT ( 'NONE',  ( 184.8333333333333144, 6.668395609140177704, -3.849999999999998312 ) ) ;
#129021=CARTESIAN_POINT ( 'NONE',  ( 184.8177083336747160, 4.367472073101515306, 7.564683531250000925 ) ) ;
#129096=CYLINDRICAL_SURFACE ( 'NONE', #62691, 7.699999999999999289 ) ;
#129144=CARTESIAN_POINT ( 'NONE',  ( 185.7083333333333428, -4.445597072760163471, -7.699999999999919353 ) ) ;
#129187=UNCERTAINTY_MEASURE_WITH_UNIT (LENGTH_MEASURE( 1.000000000000000082E-05 ), #57700, 'distance_accuracy_value', 'NONE');
#129199=CARTESIAN_POINT ( 'NONE',  ( 186.2812500006828031, 0.000000000000000000, 7.700000000000000178 ) ) ;
#129551=EDGE_CURVE ( 'NONE', #117178, #97440, #14229, .T. ) ;
#129608=CARTESIAN_POINT ( 'NONE',  ( 184.5000000000000000, 0.000000000000000000, -7.699999999999999289 ) ) ;
#129617=CARTESIAN_POINT ( 'NONE',  ( 184.5000000000000000, 0.000000000000000000, 7.700000000000000178 ) ) ;
ENDSEC;
END-ISO-10303-21;
